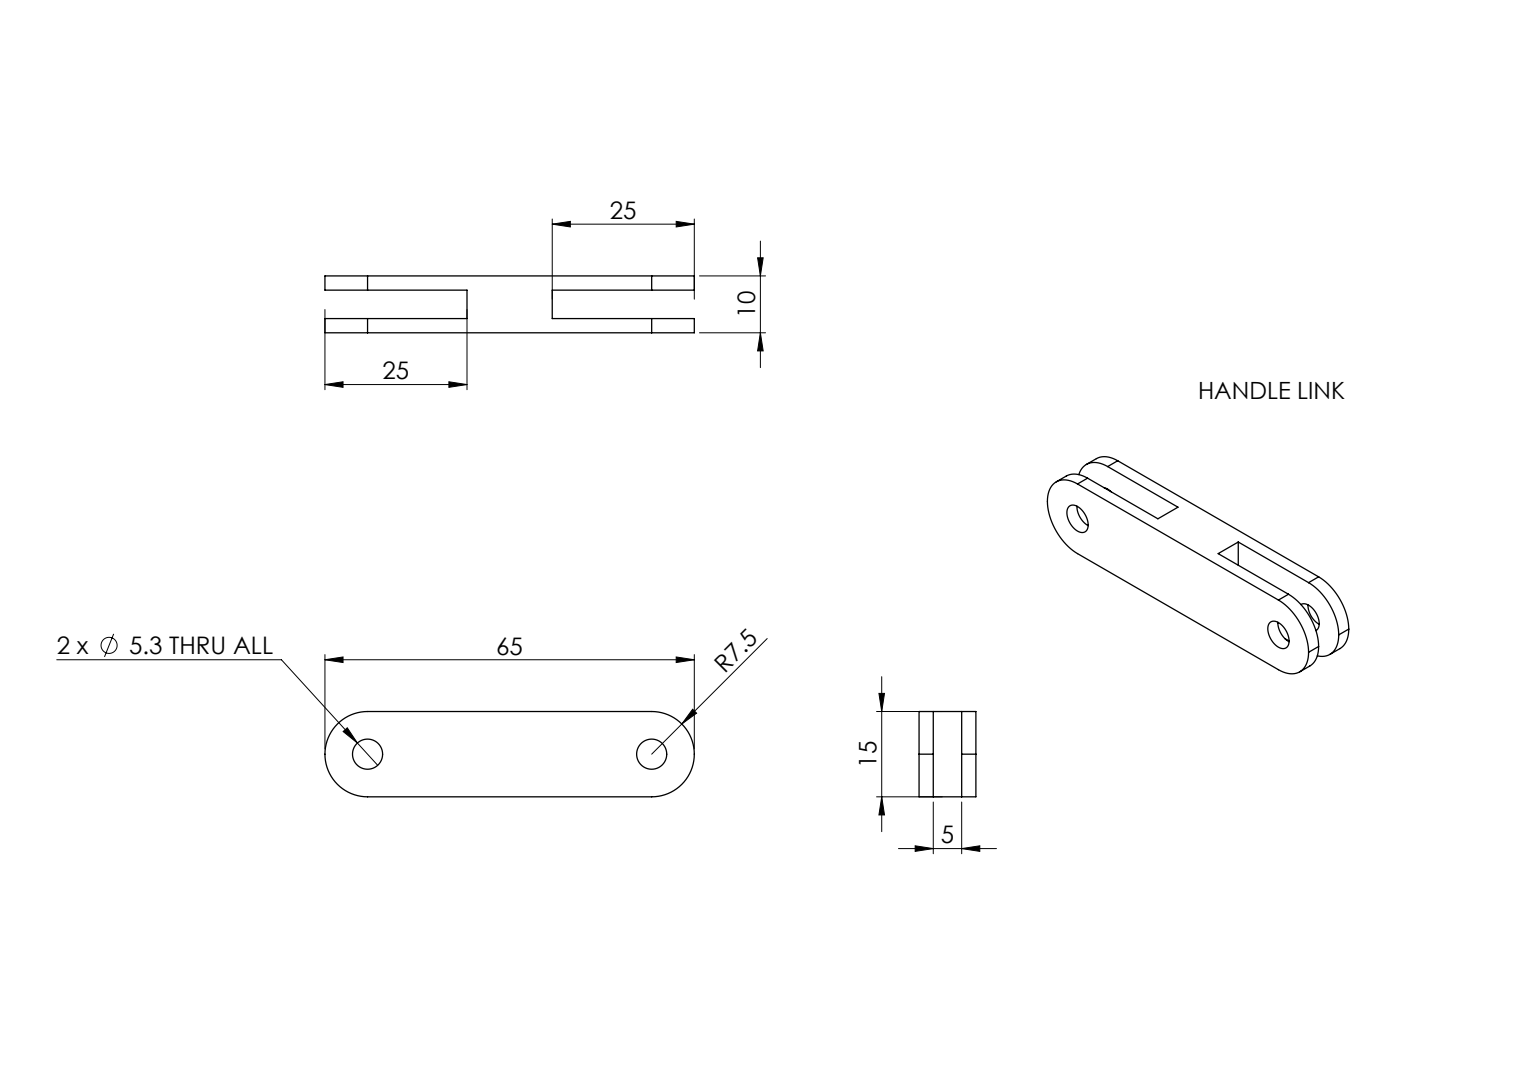
ISO-10303-21;
HEADER;
FILE_DESCRIPTION (('STEP AP214'),
    '1' );
FILE_NAME ('handle link.step',
    '2026-10-31T03:36:27',
    ( '' ),
    ( '' ),
    'SwSTEP 2.0',
    'SolidWorks 2026',
    '' );
FILE_SCHEMA (( 'AUTOMOTIVE_DESIGN' ));
ENDSEC;

DATA;
#3=ORIENTED_EDGE ( 'NONE', *, *, #2176, .T. ) ;
#65=ORIENTED_EDGE ( 'NONE', *, *, #28486, .T. ) ;
#85=DIRECTION ( 'NONE',  ( -0.000000000000000000, -0.000000000000000000, 1.000000000000000000 ) ) ;
#238=DIRECTION ( 'NONE',  ( -0.000000000000000000, -0.000000000000000000, 1.000000000000000000 ) ) ;
#278=CARTESIAN_POINT ( 'NONE',  ( -44.35000000000001563, 244.5000000000000000, -5.000000000000001776 ) ) ;
#331=DIRECTION ( 'NONE',  ( 0.000000000000000000, -0.000000000000000000, -1.000000000000000000 ) ) ;
#370=FACE_BOUND ( 'NONE', #668, .T. ) ;
#371=CARTESIAN_POINT ( 'NONE',  ( 0.3500000000000065281, 244.5000000000000000, 2.500000000000000000 ) ) ;
#373=DIRECTION ( 'NONE',  ( 0.000000000000000000, 0.000000000000000000, -1.000000000000000000 ) ) ;
#397=ORIENTED_EDGE ( 'NONE', *, *, #22014, .F. ) ;
#412=EDGE_CURVE ( 'NONE', #35111, #30074, #26288, .T. ) ;
#462=CIRCLE ( 'NONE', #24693, 2.649999999999992806 ) ;
#468=CARTESIAN_POINT ( 'NONE',  ( -54.50000000000000711, 244.5000000000000000, 5.000000000000000000 ) ) ;
#507=CARTESIAN_POINT ( 'NONE',  ( -47.00000000000000711, 244.5000000000000000, 5.000000000000000000 ) ) ;
#561=ORIENTED_EDGE ( 'NONE', *, *, #19014, .T. ) ;
#607=LINE ( 'NONE', #12176, #4334 ) ;
#668=EDGE_LOOP ( 'NONE', ( #20169, #31323 ) ) ;
#707=CIRCLE ( 'NONE', #4958, 2.649999999999991029 ) ;
#709=CARTESIAN_POINT ( 'NONE',  ( -49.64999999999999858, 244.5000000000000000, 5.000000000000000000 ) ) ;
#746=EDGE_CURVE ( 'NONE', #7363, #18087, #6969, .T. ) ;
#783=ORIENTED_EDGE ( 'NONE', *, *, #9463, .T. ) ;
#801=DIRECTION ( 'NONE',  ( 1.000000000000000000, 0.000000000000000000, 0.000000000000000000 ) ) ;
#814=CIRCLE ( 'NONE', #21430, 7.500000000000000000 ) ;
#882=ORIENTED_EDGE ( 'NONE', *, *, #5987, .T. ) ;
#914=LINE ( 'NONE', #15712, #11994 ) ;
#970=DIRECTION ( 'NONE',  ( -0.000000000000000000, -0.000000000000000000, 1.000000000000000000 ) ) ;
#1013=EDGE_CURVE ( 'NONE', #2263, #13555, #35585, .T. ) ;
#1029=LINE ( 'NONE', #4436, #15658 ) ;
#1046=ORIENTED_EDGE ( 'NONE', *, *, #23097, .F. ) ;
#1099=ORIENTED_EDGE ( 'NONE', *, *, #4077, .T. ) ;
#1123=CARTESIAN_POINT ( 'NONE',  ( 10.49999999999999645, 252.0000000000000000, -2.499999999999999556 ) ) ;
#1162=ORIENTED_EDGE ( 'NONE', *, *, #2683, .T. ) ;
#1167=DIRECTION ( 'NONE',  ( -0.000000000000000000, 1.000000000000000000, -0.000000000000000000 ) ) ;
#1216=FACE_OUTER_BOUND ( 'NONE', #2406, .T. ) ;
#1222=ORIENTED_EDGE ( 'NONE', *, *, #25857, .T. ) ;
#1245=FACE_OUTER_BOUND ( 'NONE', #30744, .T. ) ;
#1273=FACE_OUTER_BOUND ( 'NONE', #14565, .T. ) ;
#1385=VECTOR ( 'NONE', #16289, 1000.000000000000000 ) ;
#1454=CIRCLE ( 'NONE', #28104, 2.649999999999991029 ) ;
#1465=CARTESIAN_POINT ( 'NONE',  ( 2.999999999999997335, 244.5000000000000000, -2.499999999999999556 ) ) ;
#1472=CARTESIAN_POINT ( 'NONE',  ( 2.999999999999997335, 237.0000000000000000, 5.000000000000000000 ) ) ;
#1495=DIRECTION ( 'NONE',  ( 1.000000000000000000, 0.000000000000000000, 2.057406622567553763E-16 ) ) ;
#1510=CARTESIAN_POINT ( 'NONE',  ( 10.49999999999999467, 237.0000000000000000, -2.500000000000000000 ) ) ;
#1587=AXIS2_PLACEMENT_3D ( 'NONE', #16076, #33314, #36516 ) ;
#1637=ORIENTED_EDGE ( 'NONE', *, *, #15360, .F. ) ;
#1727=EDGE_LOOP ( 'NONE', ( #26472, #2358, #397, #19028 ) ) ;
#1742=CARTESIAN_POINT ( 'NONE',  ( -49.64999999999999147, 244.5000000000000000, 5.000000000000000888 ) ) ;
#1811=AXIS2_PLACEMENT_3D ( 'NONE', #26939, #970, #24112 ) ;
#1841=ORIENTED_EDGE ( 'NONE', *, *, #12878, .F. ) ;
#1883=LINE ( 'NONE', #4026, #2516 ) ;
#1921=( NAMED_UNIT ( * ) SI_UNIT ( $, .STERADIAN. ) SOLID_ANGLE_UNIT ( ) );
#1938=ORIENTED_EDGE ( 'NONE', *, *, #7640, .T. ) ;
#1964=CARTESIAN_POINT ( 'NONE',  ( -29.50000000000000711, 237.0000000000000000, -2.499999999999994671 ) ) ;
#1981=ORIENTED_EDGE ( 'NONE', *, *, #16185, .F. ) ;
#2017=CARTESIAN_POINT ( 'NONE',  ( -44.35000000000001563, 244.5000000000000000, 2.500000000000002220 ) ) ;
#2051=ADVANCED_FACE ( 'NONE', ( #370, #18586 ), #32779, .F. ) ;
#2131=LINE ( 'NONE', #10852, #3467 ) ;
#2150=LINE ( 'NONE', #1964, #13540 ) ;
#2175=CARTESIAN_POINT ( 'NONE',  ( 0.000000000000000000, 0.000000000000000000, 5.000000000000000000 ) ) ;
#2176=EDGE_CURVE ( 'NONE', #26234, #22829, #20863, .T. ) ;
#2188=EDGE_CURVE ( 'NONE', #6071, #13579, #21881, .T. ) ;
#2221=CARTESIAN_POINT ( 'NONE',  ( 10.49999999999999645, 252.0000000000000000, 2.500000000000000000 ) ) ;
#2263=VERTEX_POINT ( 'NONE', #3405 ) ;
#2308=ADVANCED_FACE ( 'NONE', ( #24627 ), #13071, .T. ) ;
#2330=FACE_OUTER_BOUND ( 'NONE', #20588, .T. ) ;
#2338=ORIENTED_EDGE ( 'NONE', *, *, #13660, .T. ) ;
#2358=ORIENTED_EDGE ( 'NONE', *, *, #23097, .T. ) ;
#2403=LINE ( 'NONE', #34432, #8203 ) ;
#2406=EDGE_LOOP ( 'NONE', ( #8339, #18616, #28272, #15794 ) ) ;
#2449=ORIENTED_EDGE ( 'NONE', *, *, #3200, .F. ) ;
#2509=CARTESIAN_POINT ( 'NONE',  ( 2.999999999999997335, 244.5000000000000000, 5.000000000000000000 ) ) ;
#2516=VECTOR ( 'NONE', #35484, 1000.000000000000000 ) ;
#2521=CARTESIAN_POINT ( 'NONE',  ( -14.50000000000000533, 237.0000000000000000, 2.500000000000000000 ) ) ;
#2546=ORIENTED_EDGE ( 'NONE', *, *, #30573, .F. ) ;
#2553=PLANE ( 'NONE',  #22436 ) ;
#2591=ORIENTED_EDGE ( 'NONE', *, *, #11969, .F. ) ;
#2625=CARTESIAN_POINT ( 'NONE',  ( -49.64999999999999858, 244.5000000000000000, -5.000000000000001776 ) ) ;
#2630=EDGE_LOOP ( 'NONE', ( #9394, #2897, #16899, #8425 ) ) ;
#2670=DIRECTION ( 'NONE',  ( 1.000000000000000000, 0.000000000000000000, 0.000000000000000000 ) ) ;
#2683=EDGE_CURVE ( 'NONE', #6822, #28262, #9292, .T. ) ;
#2705=DIRECTION ( 'NONE',  ( -1.000000000000000000, 0.000000000000000000, 0.000000000000000000 ) ) ;
#2707=ADVANCED_FACE ( 'NONE', ( #11238, #6257, #19795 ), #37195, .F. ) ;
#2831=VECTOR ( 'NONE', #373, 1000.000000000000000 ) ;
#2837=CARTESIAN_POINT ( 'NONE',  ( 2.999999999999997335, 237.0000000000000000, -5.000000000000000000 ) ) ;
#2875=ORIENTED_EDGE ( 'NONE', *, *, #11274, .F. ) ;
#2884=ORIENTED_EDGE ( 'NONE', *, *, #37146, .F. ) ;
#2897=ORIENTED_EDGE ( 'NONE', *, *, #6855, .F. ) ;
#2911=ORIENTED_EDGE ( 'NONE', *, *, #35826, .T. ) ;
#3007=ORIENTED_EDGE ( 'NONE', *, *, #16185, .T. ) ;
#3034=AXIS2_PLACEMENT_3D ( 'NONE', #30127, #4159, #1495 ) ;
#3054=ORIENTED_EDGE ( 'NONE', *, *, #7744, .T. ) ;
#3140=CARTESIAN_POINT ( 'NONE',  ( 5.649999999999991473, 244.5000000000000000, -5.000000000000001776 ) ) ;
#3174=LINE ( 'NONE', #11895, #3762 ) ;
#3191=ORIENTED_EDGE ( 'NONE', *, *, #13578, .T. ) ;
#3195=CIRCLE ( 'NONE', #34074, 2.649999999999992806 ) ;
#3200=EDGE_CURVE ( 'NONE', #9774, #8415, #9802, .T. ) ;
#3289=LINE ( 'NONE', #29442, #15484 ) ;
#3301=DIRECTION ( 'NONE',  ( 0.000000000000000000, 0.000000000000000000, -1.000000000000000000 ) ) ;
#3397=DIRECTION ( 'NONE',  ( -0.000000000000000000, -0.000000000000000000, 1.000000000000000000 ) ) ;
#3405=CARTESIAN_POINT ( 'NONE',  ( 5.649999999999985256, 244.5000000000000000, 5.000000000000000888 ) ) ;
#3467=VECTOR ( 'NONE', #11039, 1000.000000000000000 ) ;
#3543=EDGE_CURVE ( 'NONE', #22652, #25991, #3174, .T. ) ;
#3557=DIRECTION ( 'NONE',  ( 0.000000000000000000, -0.000000000000000000, -1.000000000000000000 ) ) ;
#3558=LINE ( 'NONE', #29135, #34671 ) ;
#3565=LINE ( 'NONE', #15128, #12722 ) ;
#3597=DIRECTION ( 'NONE',  ( 1.000000000000000000, 0.000000000000000000, 0.000000000000000000 ) ) ;
#3698=VERTEX_POINT ( 'NONE', #29326 ) ;
#3710=CARTESIAN_POINT ( 'NONE',  ( -47.00000000000000711, 237.0000000000000000, -5.000000000000000000 ) ) ;
#3718=CARTESIAN_POINT ( 'NONE',  ( -47.00000000000000711, 244.5000000000000000, 5.000000000000000000 ) ) ;
#3737=CARTESIAN_POINT ( 'NONE',  ( 2.999999999999997335, 244.5000000000000000, -2.499999999999999556 ) ) ;
#3762=VECTOR ( 'NONE', #35017, 1000.000000000000000 ) ;
#3778=DIRECTION ( 'NONE',  ( -1.000000000000000000, 0.000000000000000000, -0.000000000000000000 ) ) ;
#3907=CYLINDRICAL_SURFACE ( 'NONE', #14357, 2.649999999999992806 ) ;
#3929=CARTESIAN_POINT ( 'NONE',  ( -14.50000000000000533, 237.0000000000000000, 2.500000000000000000 ) ) ;
#3945=ORIENTED_EDGE ( 'NONE', *, *, #11087, .F. ) ;
#4026=CARTESIAN_POINT ( 'NONE',  ( 10.49999999999999645, 252.0000000000000000, 5.000000000000000000 ) ) ;
#4065=EDGE_CURVE ( 'NONE', #20125, #23018, #707, .T. ) ;
#4077=EDGE_CURVE ( 'NONE', #26234, #30347, #12463, .T. ) ;
#4138=ORIENTED_EDGE ( 'NONE', *, *, #3543, .T. ) ;
#4156=CARTESIAN_POINT ( 'NONE',  ( -47.00000000000000711, 244.5000000000000000, -2.499999999999997780 ) ) ;
#4159=DIRECTION ( 'NONE',  ( -2.057406622567553763E-16, 0.000000000000000000, 1.000000000000000000 ) ) ;
#4167=ORIENTED_EDGE ( 'NONE', *, *, #17535, .T. ) ;
#4206=FACE_OUTER_BOUND ( 'NONE', #5940, .T. ) ;
#4216=EDGE_LOOP ( 'NONE', ( #33261, #19684 ) ) ;
#4281=DIRECTION ( 'NONE',  ( -0.000000000000000000, -0.000000000000000000, 1.000000000000000000 ) ) ;
#4334=VECTOR ( 'NONE', #23750, 1000.000000000000000 ) ;
#4337=DIRECTION ( 'NONE',  ( 0.000000000000000000, 0.000000000000000000, -1.000000000000000000 ) ) ;
#4418=SHAPE_REPRESENTATION_RELATIONSHIP ( 'NONE' , 'NONE' ,  #16167, #5631 ) ;
#4436=CARTESIAN_POINT ( 'NONE',  ( -44.35000000000001563, 244.5000000000000000, 5.000000000000000000 ) ) ;
#4651=DIRECTION ( 'NONE',  ( 0.000000000000000000, 0.000000000000000000, 1.000000000000000000 ) ) ;
#4680=DIRECTION ( 'NONE',  ( 1.000000000000000000, 0.000000000000000000, 0.000000000000000000 ) ) ;
#4701=DIRECTION ( 'NONE',  ( 1.000000000000000000, 0.000000000000000000, 0.000000000000000000 ) ) ;
#4709=CARTESIAN_POINT ( 'NONE',  ( -14.50000000000000533, 237.0000000000000000, -2.500000000000000000 ) ) ;
#4714=AXIS2_PLACEMENT_3D ( 'NONE', #16980, #85, #37056 ) ;
#4765=AXIS2_PLACEMENT_3D ( 'NONE', #507, #31982, #5827 ) ;
#4839=CIRCLE ( 'NONE', #1811, 2.649999999999987477 ) ;
#4862=CARTESIAN_POINT ( 'NONE',  ( 0.3500000000000030864, 244.5000000000000000, -5.000000000000001776 ) ) ;
#4879=EDGE_LOOP ( 'NONE', ( #1046, #2449, #7578, #23453 ) ) ;
#4910=DIRECTION ( 'NONE',  ( -0.000000000000000000, -0.000000000000000000, 1.000000000000000000 ) ) ;
#4923=CARTESIAN_POINT ( 'NONE',  ( -29.50000000000000711, 252.0000000000000000, 5.000000000000000000 ) ) ;
#4937=CARTESIAN_POINT ( 'NONE',  ( -54.50000000000000711, 244.5000000000000000, -5.000000000000000000 ) ) ;
#4958=AXIS2_PLACEMENT_3D ( 'NONE', #3737, #3557, #15310 ) ;
#5133=LINE ( 'NONE', #19755, #11840 ) ;
#5159=PRESENTATION_STYLE_ASSIGNMENT (( #36626 ) ) ;
#5172=EDGE_CURVE ( 'NONE', #16919, #9886, #2150, .T. ) ;
#5199=EDGE_LOOP ( 'NONE', ( #10198, #34656, #29786, #28896 ) ) ;
#5275=CYLINDRICAL_SURFACE ( 'NONE', #14283, 2.649999999999992806 ) ;
#5328=LINE ( 'NONE', #11204, #35424 ) ;
#5352=CIRCLE ( 'NONE', #18095, 7.500000000000000000 ) ;
#5631=ADVANCED_BREP_SHAPE_REPRESENTATION ( '', ( #20231, #17215 ), #9874 ) ;
#5674=EDGE_CURVE ( 'NONE', #22116, #2263, #17878, .T. ) ;
#5688=CIRCLE ( 'NONE', #33550, 7.500000000000000000 ) ;
#5696=CARTESIAN_POINT ( 'NONE',  ( -47.00000000000000711, 244.5000000000000000, 2.500000000000001776 ) ) ;
#5734=DIRECTION ( 'NONE',  ( 0.000000000000000000, 0.000000000000000000, -1.000000000000000000 ) ) ;
#5827=DIRECTION ( 'NONE',  ( 1.000000000000000000, 0.000000000000000000, 0.000000000000000000 ) ) ;
#5877=ORIENTED_EDGE ( 'NONE', *, *, #30573, .T. ) ;
#5927=CIRCLE ( 'NONE', #9568, 7.500000000000000000 ) ;
#5940=EDGE_LOOP ( 'NONE', ( #8655, #3007, #28913, #16752 ) ) ;
#5961=EDGE_LOOP ( 'NONE', ( #12843, #35401, #13130, #13842 ) ) ;
#5987=EDGE_CURVE ( 'NONE', #22652, #8155, #814, .T. ) ;
#5990=EDGE_LOOP ( 'NONE', ( #24725, #23324 ) ) ;
#6018=FACE_OUTER_BOUND ( 'NONE', #27165, .T. ) ;
#6071=VERTEX_POINT ( 'NONE', #1742 ) ;
#6157=EDGE_CURVE ( 'NONE', #22829, #3698, #5328, .T. ) ;
#6253=DIRECTION ( 'NONE',  ( -0.000000000000000000, -0.000000000000000000, 1.000000000000000000 ) ) ;
#6257=FACE_BOUND ( 'NONE', #4216, .T. ) ;
#6346=EDGE_CURVE ( 'NONE', #37113, #27676, #28190, .T. ) ;
#6491=ORIENTED_EDGE ( 'NONE', *, *, #17296, .T. ) ;
#6492=CARTESIAN_POINT ( 'NONE',  ( 2.999999999999997335, 244.5000000000000000, 5.000000000000000000 ) ) ;
#6497=CARTESIAN_POINT ( 'NONE',  ( 5.649999999999987921, 244.5000000000000000, 5.000000000000000000 ) ) ;
#6522=( LENGTH_UNIT ( ) NAMED_UNIT ( * ) SI_UNIT ( .MILLI., .METRE. ) );
#6700=ORIENTED_EDGE ( 'NONE', *, *, #35373, .F. ) ;
#6773=DIRECTION ( 'NONE',  ( 0.000000000000000000, 0.000000000000000000, 1.000000000000000000 ) ) ;
#6796=EDGE_CURVE ( 'NONE', #8155, #18512, #36709, .T. ) ;
#6814=CARTESIAN_POINT ( 'NONE',  ( -47.00000000000000711, 244.5000000000000000, 5.000000000000000888 ) ) ;
#6822=VERTEX_POINT ( 'NONE', #17374 ) ;
#6855=EDGE_CURVE ( 'NONE', #19498, #35111, #14874, .T. ) ;
#6872=STYLED_ITEM ( 'NONE', ( #5159 ), #5631 ) ;
#6900=( NAMED_UNIT ( * ) PLANE_ANGLE_UNIT ( ) SI_UNIT ( $, .RADIAN. ) );
#6947=CARTESIAN_POINT ( 'NONE',  ( -47.00000000000000711, 244.5000000000000000, -2.499999999999997780 ) ) ;
#6969=LINE ( 'NONE', #24759, #12914 ) ;
#6988=DIRECTION ( 'NONE',  ( -0.000000000000000000, -0.000000000000000000, 1.000000000000000000 ) ) ;
#7001=CIRCLE ( 'NONE', #17894, 7.500000000000000000 ) ;
#7062=AXIS2_PLACEMENT_3D ( 'NONE', #31879, #19787, #8763 ) ;
#7110=VECTOR ( 'NONE', #36576, 1000.000000000000000 ) ;
#7176=CARTESIAN_POINT ( 'NONE',  ( 2.999999999999997335, 252.0000000000000000, -2.499999999999999556 ) ) ;
#7252=LINE ( 'NONE', #32828, #16365 ) ;
#7255=DIRECTION ( 'NONE',  ( 1.000000000000000000, 0.000000000000000000, 0.000000000000000000 ) ) ;
#7303=CARTESIAN_POINT ( 'NONE',  ( -54.50000000000000711, 244.5000000000000000, -2.499999999999996003 ) ) ;
#7315=DIRECTION ( 'NONE',  ( 1.000000000000000000, 0.000000000000000000, 1.636531581110199847E-16 ) ) ;
#7320=DIRECTION ( 'NONE',  ( -2.057406622567553763E-16, 0.000000000000000000, 1.000000000000000000 ) ) ;
#7354=CYLINDRICAL_SURFACE ( 'NONE', #21587, 2.649999999999991029 ) ;
#7363=VERTEX_POINT ( 'NONE', #32503 ) ;
#7364=VECTOR ( 'NONE', #35617, 1000.000000000000000 ) ;
#7379=AXIS2_PLACEMENT_3D ( 'NONE', #24131, #4910, #801 ) ;
#7529=AXIS2_PLACEMENT_3D ( 'NONE', #20789, #9780, #12624 ) ;
#7541=DIRECTION ( 'NONE',  ( -1.000000000000000000, 0.000000000000000000, 0.000000000000000000 ) ) ;
#7578=ORIENTED_EDGE ( 'NONE', *, *, #20721, .T. ) ;
#7588=CIRCLE ( 'NONE', #34813, 2.649999999999992806 ) ;
#7623=( LENGTH_UNIT ( ) NAMED_UNIT ( * ) SI_UNIT ( .MILLI., .METRE. ) );
#7640=EDGE_CURVE ( 'NONE', #22958, #37113, #5688, .T. ) ;
#7744=EDGE_CURVE ( 'NONE', #9886, #19776, #29044, .T. ) ;
#7861=LINE ( 'NONE', #30983, #27840 ) ;
#7973=AXIS2_PLACEMENT_3D ( 'NONE', #28857, #238, #14843 ) ;
#8154=EDGE_LOOP ( 'NONE', ( #28821, #2546, #20599, #10061, #36654 ) ) ;
#8155=VERTEX_POINT ( 'NONE', #2837 ) ;
#8174=DIRECTION ( 'NONE',  ( 0.000000000000000000, 0.000000000000000000, 1.000000000000000000 ) ) ;
#8203=VECTOR ( 'NONE', #29101, 1000.000000000000000 ) ;
#8279=DIRECTION ( 'NONE',  ( -1.000000000000000000, 0.000000000000000000, 0.000000000000000000 ) ) ;
#8299=EDGE_CURVE ( 'NONE', #18605, #13555, #34233, .T. ) ;
#8339=ORIENTED_EDGE ( 'NONE', *, *, #19918, .F. ) ;
#8341=CARTESIAN_POINT ( 'NONE',  ( 10.49999999999999467, 237.0000000000000000, -2.500000000000000000 ) ) ;
#8375=DIRECTION ( 'NONE',  ( -0.000000000000000000, -0.000000000000000000, 1.000000000000000000 ) ) ;
#8395=VERTEX_POINT ( 'NONE', #2017 ) ;
#8415=VERTEX_POINT ( 'NONE', #4862 ) ;
#8425=ORIENTED_EDGE ( 'NONE', *, *, #25413, .T. ) ;
#8464=DIRECTION ( 'NONE',  ( -0.000000000000000000, -0.000000000000000000, 1.000000000000000000 ) ) ;
#8536=CARTESIAN_POINT ( 'NONE',  ( 2.999999999999997335, 252.0000000000000000, 5.000000000000000000 ) ) ;
#8545=EDGE_LOOP ( 'NONE', ( #21634, #17320, #12168, #8842 ) ) ;
#8594=VERTEX_POINT ( 'NONE', #468 ) ;
#8655=ORIENTED_EDGE ( 'NONE', *, *, #31634, .F. ) ;
#8763=DIRECTION ( 'NONE',  ( -1.000000000000000000, 0.000000000000000000, 0.000000000000000000 ) ) ;
#8778=CARTESIAN_POINT ( 'NONE',  ( 2.999999999999997335, 244.5000000000000000, 5.000000000000000000 ) ) ;
#8786=CARTESIAN_POINT ( 'NONE',  ( 2.999999999999997335, 244.5000000000000000, 5.000000000000000000 ) ) ;
#8797=ORIENTED_EDGE ( 'NONE', *, *, #9372, .F. ) ;
#8800=FACE_OUTER_BOUND ( 'NONE', #5199, .T. ) ;
#8842=ORIENTED_EDGE ( 'NONE', *, *, #25857, .F. ) ;
#8902=ADVANCED_FACE ( 'NONE', ( #1216 ), #12983, .T. ) ;
#8907=AXIS2_PLACEMENT_3D ( 'NONE', #21819, #22562, #28052 ) ;
#9029=DIRECTION ( 'NONE',  ( -1.000000000000000000, -0.000000000000000000, -0.000000000000000000 ) ) ;
#9107=( GEOMETRIC_REPRESENTATION_CONTEXT ( 3 ) GLOBAL_UNCERTAINTY_ASSIGNED_CONTEXT ( ( #30949 ) ) GLOBAL_UNIT_ASSIGNED_CONTEXT ( ( #7623, #16529, #1921 ) ) REPRESENTATION_CONTEXT ( 'NONE', 'WORKASPACE' ) );
#9234=EDGE_CURVE ( 'NONE', #13579, #6071, #18891, .T. ) ;
#9292=LINE ( 'NONE', #2521, #2831 ) ;
#9372=EDGE_CURVE ( 'NONE', #8155, #25296, #607, .T. ) ;
#9384=ADVANCED_FACE ( 'NONE', ( #32455 ), #34735, .T. ) ;
#9394=ORIENTED_EDGE ( 'NONE', *, *, #412, .F. ) ;
#9434=LINE ( 'NONE', #29327, #32953 ) ;
#9463=EDGE_CURVE ( 'NONE', #27676, #12668, #1883, .T. ) ;
#9509=ADVANCED_FACE ( 'NONE', ( #24320 ), #12565, .F. ) ;
#9528=DIRECTION ( 'NONE',  ( 0.000000000000000000, 0.000000000000000000, -1.000000000000000000 ) ) ;
#9534=CARTESIAN_POINT ( 'NONE',  ( -44.35000000000001563, 244.5000000000000000, -2.499999999999997335 ) ) ;
#9568=AXIS2_PLACEMENT_3D ( 'NONE', #33173, #16493, #25006 ) ;
#9774=VERTEX_POINT ( 'NONE', #3140 ) ;
#9780=DIRECTION ( 'NONE',  ( 2.057406622567553763E-16, -0.000000000000000000, -1.000000000000000000 ) ) ;
#9802=CIRCLE ( 'NONE', #18915, 2.649999999999994582 ) ;
#9814=CARTESIAN_POINT ( 'NONE',  ( -49.64999999999999858, 244.5000000000000000, 2.500000000000001332 ) ) ;
#9874=( GEOMETRIC_REPRESENTATION_CONTEXT ( 3 ) GLOBAL_UNCERTAINTY_ASSIGNED_CONTEXT ( ( #30177 ) ) GLOBAL_UNIT_ASSIGNED_CONTEXT ( ( #6522, #6900, #26793 ) ) REPRESENTATION_CONTEXT ( 'NONE', 'WORKASPACE' ) );
#9886=VERTEX_POINT ( 'NONE', #36279 ) ;
#9963=DIRECTION ( 'NONE',  ( -2.057406622567553763E-16, 0.000000000000000000, 1.000000000000000000 ) ) ;
#9964=CARTESIAN_POINT ( 'NONE',  ( -54.50000000000000711, 244.5000000000000000, 2.500000000000000000 ) ) ;
#9998=CARTESIAN_POINT ( 'NONE',  ( 2.999999999999997335, 244.5000000000000000, -5.000000000000000000 ) ) ;
#10061=ORIENTED_EDGE ( 'NONE', *, *, #11969, .T. ) ;
#10109=ADVANCED_FACE ( 'NONE', ( #30533, #28786 ), #26640, .F. ) ;
#10126=EDGE_LOOP ( 'NONE', ( #37387, #24919, #12050, #3054 ) ) ;
#10188=ORIENTED_EDGE ( 'NONE', *, *, #5172, .F. ) ;
#10198=ORIENTED_EDGE ( 'NONE', *, *, #8299, .F. ) ;
#10201=PRODUCT_DEFINITION ( 'UNKNOWN', '', #22055, #26269 ) ;
#10259=EDGE_LOOP ( 'NONE', ( #16320, #36183, #33664, #12933 ) ) ;
#10274=CARTESIAN_POINT ( 'NONE',  ( 2.999999999999997335, 244.5000000000000000, -5.000000000000000000 ) ) ;
#10343=CARTESIAN_POINT ( 'NONE',  ( -47.00000000000000711, 244.5000000000000000, 2.500000000000001776 ) ) ;
#10463=DIRECTION ( 'NONE',  ( 1.000000000000000000, 0.000000000000000000, 0.000000000000000000 ) ) ;
#10464=EDGE_LOOP ( 'NONE', ( #10725, #31213, #2875, #18973 ) ) ;
#10501=VECTOR ( 'NONE', #18451, 1000.000000000000000 ) ;
#10560=DIRECTION ( 'NONE',  ( 0.000000000000000000, -0.000000000000000000, -1.000000000000000000 ) ) ;
#10620=ORIENTED_EDGE ( 'NONE', *, *, #14204, .T. ) ;
#10647=CARTESIAN_POINT ( 'NONE',  ( -47.00000000000000711, 244.5000000000000000, -5.000000000000001776 ) ) ;
#10665=( LENGTH_UNIT ( ) NAMED_UNIT ( * ) SI_UNIT ( .MILLI., .METRE. ) );
#10704=ORIENTED_EDGE ( 'NONE', *, *, #412, .T. ) ;
#10725=ORIENTED_EDGE ( 'NONE', *, *, #24289, .F. ) ;
#10779=ADVANCED_FACE ( 'NONE', ( #33119 ), #18350, .T. ) ;
#10821=CYLINDRICAL_SURFACE ( 'NONE', #24614, 7.500000000000000000 ) ;
#10852=CARTESIAN_POINT ( 'NONE',  ( 10.49999999999999645, 252.0000000000000000, 2.500000000000013323 ) ) ;
#10853=( NAMED_UNIT ( * ) SI_UNIT ( $, .STERADIAN. ) SOLID_ANGLE_UNIT ( ) );
#10934=CARTESIAN_POINT ( 'NONE',  ( 2.999999999999997335, 237.0000000000000000, 5.000000000000000000 ) ) ;
#10935=AXIS2_PLACEMENT_3D ( 'NONE', #10343, #7320, #18521 ) ;
#10991=EDGE_CURVE ( 'NONE', #30074, #14298, #3195, .T. ) ;
#11006=CARTESIAN_POINT ( 'NONE',  ( -47.00000000000000711, 244.5000000000000000, 5.000000000000000000 ) ) ;
#11008=ADVANCED_FACE ( 'NONE', ( #27276 ), #35613, .T. ) ;
#11039=DIRECTION ( 'NONE',  ( -1.000000000000000000, 0.000000000000000000, -2.057406622567553763E-16 ) ) ;
#11068=DIRECTION ( 'NONE',  ( 1.000000000000000000, 0.000000000000000000, 2.057406622567553516E-16 ) ) ;
#11087=EDGE_CURVE ( 'NONE', #28262, #26234, #30692, .T. ) ;
#11115=CARTESIAN_POINT ( 'NONE',  ( -29.50000000000000711, 237.0000000000000000, -2.499999999999994671 ) ) ;
#11189=FACE_OUTER_BOUND ( 'NONE', #8545, .T. ) ;
#11204=CARTESIAN_POINT ( 'NONE',  ( 2.999999999999997335, 252.0000000000000000, -5.000000000000000000 ) ) ;
#11238=FACE_BOUND ( 'NONE', #18843, .T. ) ;
#11266=ORIENTED_EDGE ( 'NONE', *, *, #746, .T. ) ;
#11274=EDGE_CURVE ( 'NONE', #8594, #36846, #5352, .T. ) ;
#11293=CARTESIAN_POINT ( 'NONE',  ( -54.50000000000000711, 237.0000000000000000, -2.500000000000000000 ) ) ;
#11434=DIRECTION ( 'NONE',  ( -1.000000000000000000, 0.000000000000000000, -0.000000000000000000 ) ) ;
#11488=ORIENTED_EDGE ( 'NONE', *, *, #19918, .T. ) ;
#11511=AXIS2_PLACEMENT_3D ( 'NONE', #25828, #14459, #26014 ) ;
#11527=DIRECTION ( 'NONE',  ( 0.000000000000000000, -1.000000000000000000, 0.000000000000000000 ) ) ;
#11552=EDGE_CURVE ( 'NONE', #12668, #8594, #27770, .T. ) ;
#11840=VECTOR ( 'NONE', #34683, 1000.000000000000000 ) ;
#11895=CARTESIAN_POINT ( 'NONE',  ( 10.49999999999999645, 244.5000000000000000, 5.000000000000000000 ) ) ;
#11907=DIRECTION ( 'NONE',  ( -1.000000000000000000, 0.000000000000000000, 0.000000000000000000 ) ) ;
#11969=EDGE_CURVE ( 'NONE', #16035, #16919, #19658, .T. ) ;
#11994=VECTOR ( 'NONE', #33141, 1000.000000000000000 ) ;
#12050=ORIENTED_EDGE ( 'NONE', *, *, #5172, .T. ) ;
#12077=DIRECTION ( 'NONE',  ( -0.000000000000000000, -0.000000000000000000, 1.000000000000000000 ) ) ;
#12119=LINE ( 'NONE', #23886, #15170 ) ;
#12121=LINE ( 'NONE', #26712, #32691 ) ;
#12168=ORIENTED_EDGE ( 'NONE', *, *, #11552, .F. ) ;
#12176=CARTESIAN_POINT ( 'NONE',  ( 10.49999999999999645, 237.0000000000000000, -5.000000000000000000 ) ) ;
#12331=ORIENTED_EDGE ( 'NONE', *, *, #5987, .F. ) ;
#12463=LINE ( 'NONE', #24032, #27344 ) ;
#12497=DIRECTION ( 'NONE',  ( -1.000000000000000000, 0.000000000000000000, 0.000000000000000000 ) ) ;
#12565=CYLINDRICAL_SURFACE ( 'NONE', #7379, 2.649999999999992806 ) ;
#12624=DIRECTION ( 'NONE',  ( 1.000000000000000000, 0.000000000000000000, 2.312964634635742957E-16 ) ) ;
#12628=FACE_BOUND ( 'NONE', #5990, .T. ) ;
#12644=DIRECTION ( 'NONE',  ( -0.000000000000000000, -0.000000000000000000, 1.000000000000000000 ) ) ;
#12648=FACE_OUTER_BOUND ( 'NONE', #36783, .T. ) ;
#12668=VERTEX_POINT ( 'NONE', #30027 ) ;
#12676=CARTESIAN_POINT ( 'NONE',  ( -14.50000000000000533, 237.0000000000000000, -2.500000000000000000 ) ) ;
#12689=DIRECTION ( 'NONE',  ( 1.000000000000000000, 0.000000000000000000, 2.057406622567553763E-16 ) ) ;
#12722=VECTOR ( 'NONE', #19809, 1000.000000000000000 ) ;
#12739=CARTESIAN_POINT ( 'NONE',  ( -47.00000000000000711, 252.0000000000000000, -2.499999999999997780 ) ) ;
#12747=CIRCLE ( 'NONE', #30907, 7.500000000000000000 ) ;
#12762=CIRCLE ( 'NONE', #19462, 2.649999999999991029 ) ;
#12825=ORIENTED_EDGE ( 'NONE', *, *, #4077, .F. ) ;
#12843=ORIENTED_EDGE ( 'NONE', *, *, #37247, .F. ) ;
#12878=EDGE_CURVE ( 'NONE', #19498, #14298, #1029, .T. ) ;
#12895=AXIS2_PLACEMENT_3D ( 'NONE', #30508, #16104, #24441 ) ;
#12914=VECTOR ( 'NONE', #35943, 1000.000000000000000 ) ;
#12933=ORIENTED_EDGE ( 'NONE', *, *, #6157, .F. ) ;
#12983=CYLINDRICAL_SURFACE ( 'NONE', #13585, 7.500000000000000000 ) ;
#13070=FACE_BOUND ( 'NONE', #24873, .T. ) ;
#13071=CYLINDRICAL_SURFACE ( 'NONE', #28853, 7.500000000000000000 ) ;
#13130=ORIENTED_EDGE ( 'NONE', *, *, #35419, .F. ) ;
#13172=CARTESIAN_POINT ( 'NONE',  ( 2.999999999999997335, 244.5000000000000000, -2.499999999999999556 ) ) ;
#13247=CARTESIAN_POINT ( 'NONE',  ( 2.999999999999997335, 244.5000000000000000, -5.000000000000001776 ) ) ;
#13338=CIRCLE ( 'NONE', #34519, 7.500000000000000000 ) ;
#13376=DIRECTION ( 'NONE',  ( -0.000000000000000000, 0.000000000000000000, 1.000000000000000000 ) ) ;
#13456=FACE_OUTER_BOUND ( 'NONE', #31538, .T. ) ;
#13540=VECTOR ( 'NONE', #27934, 1000.000000000000000 ) ;
#13552=ORIENTED_EDGE ( 'NONE', *, *, #18146, .F. ) ;
#13554=ORIENTED_EDGE ( 'NONE', *, *, #2188, .T. ) ;
#13555=VERTEX_POINT ( 'NONE', #23662 ) ;
#13578=EDGE_CURVE ( 'NONE', #21882, #6071, #14942, .T. ) ;
#13579=VERTEX_POINT ( 'NONE', #21019 ) ;
#13585=AXIS2_PLACEMENT_3D ( 'NONE', #21706, #18495, #33256 ) ;
#13595=CARTESIAN_POINT ( 'NONE',  ( 0.3500000000000065281, 244.5000000000000000, 5.000000000000000000 ) ) ;
#13623=EDGE_CURVE ( 'NONE', #16919, #20032, #3565, .T. ) ;
#13660=EDGE_CURVE ( 'NONE', #36103, #9886, #7861, .T. ) ;
#13757=DIRECTION ( 'NONE',  ( 1.000000000000000000, 0.000000000000000000, 0.000000000000000000 ) ) ;
#13836=DIRECTION ( 'NONE',  ( -1.000000000000000000, -0.000000000000000000, -0.000000000000000000 ) ) ;
#13842=ORIENTED_EDGE ( 'NONE', *, *, #6346, .F. ) ;
#13877=DIRECTION ( 'NONE',  ( -0.000000000000000000, -0.000000000000000000, 1.000000000000000000 ) ) ;
#13888=EDGE_CURVE ( 'NONE', #13555, #2263, #4839, .T. ) ;
#13901=DIRECTION ( 'NONE',  ( 0.000000000000000000, -0.000000000000000000, -1.000000000000000000 ) ) ;
#13909=ORIENTED_EDGE ( 'NONE', *, *, #9234, .F. ) ;
#13933=ORIENTED_EDGE ( 'NONE', *, *, #25413, .F. ) ;
#14204=EDGE_CURVE ( 'NONE', #3698, #7363, #28487, .T. ) ;
#14283=AXIS2_PLACEMENT_3D ( 'NONE', #20816, #12077, #20628 ) ;
#14298=VERTEX_POINT ( 'NONE', #9534 ) ;
#14357=AXIS2_PLACEMENT_3D ( 'NONE', #3718, #4281, #35929 ) ;
#14459=DIRECTION ( 'NONE',  ( 0.000000000000000000, -0.000000000000000000, -1.000000000000000000 ) ) ;
#14462=DIRECTION ( 'NONE',  ( -1.000000000000000000, 0.000000000000000000, -0.000000000000000000 ) ) ;
#14474=ORIENTED_EDGE ( 'NONE', *, *, #35373, .T. ) ;
#14483=ORIENTED_EDGE ( 'NONE', *, *, #2176, .F. ) ;
#14529=ORIENTED_EDGE ( 'NONE', *, *, #9234, .T. ) ;
#14565=EDGE_LOOP ( 'NONE', ( #6491, #19954, #16359, #19403 ) ) ;
#14596=DIRECTION ( 'NONE',  ( 1.000000000000000000, 0.000000000000000000, 0.000000000000000000 ) ) ;
#14646=DIRECTION ( 'NONE',  ( 0.000000000000000000, -0.000000000000000000, -1.000000000000000000 ) ) ;
#14655=EDGE_LOOP ( 'NONE', ( #21402, #20315, #28222, #24098, #23575 ) ) ;
#14738=ORIENTED_EDGE ( 'NONE', *, *, #26044, .F. ) ;
#14782=CYLINDRICAL_SURFACE ( 'NONE', #15195, 2.649999999999991029 ) ;
#14791=DIRECTION ( 'NONE',  ( 1.000000000000000000, 0.000000000000000000, 0.000000000000000000 ) ) ;
#14843=DIRECTION ( 'NONE',  ( 1.000000000000000000, 0.000000000000000000, 0.000000000000000000 ) ) ;
#14861=CARTESIAN_POINT ( 'NONE',  ( 2.999999999999997335, 244.5000000000000000, 5.000000000000000000 ) ) ;
#14874=CIRCLE ( 'NONE', #29396, 2.649999999999992806 ) ;
#14942=LINE ( 'NONE', #709, #24810 ) ;
#14951=ORIENTED_EDGE ( 'NONE', *, *, #19014, .F. ) ;
#15034=VECTOR ( 'NONE', #35027, 1000.000000000000000 ) ;
#15128=CARTESIAN_POINT ( 'NONE',  ( -29.50000000000000711, 237.0000000000000000, -2.499999999999994671 ) ) ;
#15140=ADVANCED_FACE ( 'NONE', ( #25610 ), #34328, .T. ) ;
#15170=VECTOR ( 'NONE', #6253, 1000.000000000000000 ) ;
#15195=AXIS2_PLACEMENT_3D ( 'NONE', #22758, #3397, #37322 ) ;
#15310=DIRECTION ( 'NONE',  ( -1.000000000000000000, 0.000000000000000000, 0.000000000000000000 ) ) ;
#15311=PLANE ( 'NONE',  #19040 ) ;
#15314=CARTESIAN_POINT ( 'NONE',  ( 10.49999999999999645, 244.5000000000000000, 2.500000000000000000 ) ) ;
#15360=EDGE_CURVE ( 'NONE', #31488, #30489, #12747, .T. ) ;
#15484=VECTOR ( 'NONE', #35123, 1000.000000000000000 ) ;
#15634=AXIS2_PLACEMENT_3D ( 'NONE', #30524, #33731, #36562 ) ;
#15658=VECTOR ( 'NONE', #35527, 1000.000000000000000 ) ;
#15712=CARTESIAN_POINT ( 'NONE',  ( -47.00000000000000711, 237.0000000000000000, 5.000000000000000000 ) ) ;
#15726=DIRECTION ( 'NONE',  ( 1.000000000000000000, 0.000000000000000000, 1.636531581110199847E-16 ) ) ;
#15782=UNCERTAINTY_MEASURE_WITH_UNIT (LENGTH_MEASURE( 1.000000000000000082E-05 ), #10665, 'distance_accuracy_value', 'NONE');
#15794=ORIENTED_EDGE ( 'NONE', *, *, #19765, .F. ) ;
#15827=EDGE_CURVE ( 'NONE', #8395, #21882, #33932, .T. ) ;
#15907=ADVANCED_FACE ( 'NONE', ( #12628, #19454, #27780 ), #2553, .T. ) ;
#15970=ORIENTED_EDGE ( 'NONE', *, *, #6796, .F. ) ;
#16035=VERTEX_POINT ( 'NONE', #26794 ) ;
#16047=CARTESIAN_POINT ( 'NONE',  ( 0.000000000000000000, 0.000000000000000000, 0.000000000000000000 ) ) ;
#16076=CARTESIAN_POINT ( 'NONE',  ( 2.999999999999997335, 244.5000000000000000, 5.000000000000000000 ) ) ;
#16104=DIRECTION ( 'NONE',  ( 0.000000000000000000, 0.000000000000000000, -1.000000000000000000 ) ) ;
#16120=LINE ( 'NONE', #1510, #31968 ) ;
#16167=SHAPE_REPRESENTATION ( 'handle link', ( #17215 ), #9874 ) ;
#16185=EDGE_CURVE ( 'NONE', #30240, #31488, #13338, .T. ) ;
#16263=EDGE_LOOP ( 'NONE', ( #2911, #1637, #1981, #4167, #21374 ) ) ;
#16273=VECTOR ( 'NONE', #19127, 1000.000000000000000 ) ;
#16289=DIRECTION ( 'NONE',  ( -0.000000000000000000, 1.000000000000000000, -0.000000000000000000 ) ) ;
#16320=ORIENTED_EDGE ( 'NONE', *, *, #26959, .F. ) ;
#16359=ORIENTED_EDGE ( 'NONE', *, *, #13888, .T. ) ;
#16365=VECTOR ( 'NONE', #9528, 1000.000000000000000 ) ;
#16374=CARTESIAN_POINT ( 'NONE',  ( 2.999999999999997335, 237.0000000000000000, 2.500000000000000000 ) ) ;
#16445=PLANE ( 'NONE',  #23251 ) ;
#16480=PLANE ( 'NONE',  #3034 ) ;
#16493=DIRECTION ( 'NONE',  ( 2.057406622567553763E-16, -0.000000000000000000, -1.000000000000000000 ) ) ;
#16519=DIRECTION ( 'NONE',  ( 0.000000000000000000, 0.000000000000000000, -1.000000000000000000 ) ) ;
#16529=( NAMED_UNIT ( * ) PLANE_ANGLE_UNIT ( ) SI_UNIT ( $, .RADIAN. ) );
#16538=FACE_OUTER_BOUND ( 'NONE', #4879, .T. ) ;
#16539=ORIENTED_EDGE ( 'NONE', *, *, #23362, .F. ) ;
#16742=ORIENTED_EDGE ( 'NONE', *, *, #35419, .T. ) ;
#16752=ORIENTED_EDGE ( 'NONE', *, *, #7640, .F. ) ;
#16815=CARTESIAN_POINT ( 'NONE',  ( 2.999999999999997335, 237.0000000000000000, 5.000000000000000000 ) ) ;
#16853=DIRECTION ( 'NONE',  ( -0.000000000000000000, 0.000000000000000000, 1.000000000000000000 ) ) ;
#16899=ORIENTED_EDGE ( 'NONE', *, *, #12878, .T. ) ;
#16904=DIRECTION ( 'NONE',  ( 0.000000000000000000, 0.000000000000000000, -1.000000000000000000 ) ) ;
#16919=VERTEX_POINT ( 'NONE', #25960 ) ;
#16937=DIRECTION ( 'NONE',  ( -0.000000000000000000, 0.000000000000000000, 1.000000000000000000 ) ) ;
#16980=CARTESIAN_POINT ( 'NONE',  ( 2.999999999999997335, 244.5000000000000000, 5.000000000000000888 ) ) ;
#17064=AXIS2_PLACEMENT_3D ( 'NONE', #8778, #28668, #2705 ) ;
#17111=ADVANCED_FACE ( 'NONE', ( #17632 ), #14782, .F. ) ;
#17141=ORIENTED_EDGE ( 'NONE', *, *, #6346, .T. ) ;
#17215=AXIS2_PLACEMENT_3D ( 'NONE', #16047, #4651, #19645 ) ;
#17296=EDGE_CURVE ( 'NONE', #22116, #18605, #12762, .T. ) ;
#17320=ORIENTED_EDGE ( 'NONE', *, *, #27448, .F. ) ;
#17349=AXIS2_PLACEMENT_3D ( 'NONE', #1465, #10560, #7541 ) ;
#17374=CARTESIAN_POINT ( 'NONE',  ( -14.50000000000000533, 237.0000000000000000, 2.500000000000000000 ) ) ;
#17467=VECTOR ( 'NONE', #31201, 1000.000000000000000 ) ;
#17535=EDGE_CURVE ( 'NONE', #30240, #6822, #20227, .T. ) ;
#17632=FACE_OUTER_BOUND ( 'NONE', #1727, .T. ) ;
#17637=VECTOR ( 'NONE', #1167, 1000.000000000000000 ) ;
#17779=EDGE_LOOP ( 'NONE', ( #6700, #15970, #12331, #4138 ) ) ;
#17878=LINE ( 'NONE', #6497, #10501 ) ;
#17894=AXIS2_PLACEMENT_3D ( 'NONE', #5696, #31666, #28815 ) ;
#18016=CARTESIAN_POINT ( 'NONE',  ( -47.00000000000000711, 252.0000000000000000, 2.500000000000001776 ) ) ;
#18041=ORIENTED_EDGE ( 'NONE', *, *, #37182, .T. ) ;
#18043=ORIENTED_EDGE ( 'NONE', *, *, #6796, .T. ) ;
#18066=DIRECTION ( 'NONE',  ( 0.000000000000000000, 0.000000000000000000, -1.000000000000000000 ) ) ;
#18087=VERTEX_POINT ( 'NONE', #12739 ) ;
#18095=AXIS2_PLACEMENT_3D ( 'NONE', #25365, #33897, #37289 ) ;
#18146=EDGE_CURVE ( 'NONE', #6822, #30347, #29982, .T. ) ;
#18217=DIRECTION ( 'NONE',  ( 1.000000000000000000, 0.000000000000000000, 0.000000000000000000 ) ) ;
#18350=PLANE ( 'NONE',  #18947 ) ;
#18366=ORIENTED_EDGE ( 'NONE', *, *, #9372, .T. ) ;
#18451=DIRECTION ( 'NONE',  ( -0.000000000000000000, -0.000000000000000000, 1.000000000000000000 ) ) ;
#18474=SURFACE_STYLE_FILL_AREA ( #32852 ) ;
#18495=DIRECTION ( 'NONE',  ( 0.000000000000000000, 0.000000000000000000, -1.000000000000000000 ) ) ;
#18512=VERTEX_POINT ( 'NONE', #30560 ) ;
#18521=DIRECTION ( 'NONE',  ( 1.000000000000000000, 0.000000000000000000, 1.636531581110199847E-16 ) ) ;
#18586=FACE_OUTER_BOUND ( 'NONE', #14655, .T. ) ;
#18605=VERTEX_POINT ( 'NONE', #371 ) ;
#18616=ORIENTED_EDGE ( 'NONE', *, *, #34724, .T. ) ;
#18806=AXIS2_PLACEMENT_3D ( 'NONE', #28632, #25980, #2670 ) ;
#18843=EDGE_LOOP ( 'NONE', ( #35272, #65 ) ) ;
#18862=AXIS2_PLACEMENT_3D ( 'NONE', #26906, #27099, #12689 ) ;
#18891=CIRCLE ( 'NONE', #7973, 2.649999999999985700 ) ;
#18903=SHAPE_DEFINITION_REPRESENTATION ( #25892, #16167 ) ;
#18915=AXIS2_PLACEMENT_3D ( 'NONE', #25372, #28216, #19710 ) ;
#18947=AXIS2_PLACEMENT_3D ( 'NONE', #3929, #30313, #4337 ) ;
#18973=ORIENTED_EDGE ( 'NONE', *, *, #27448, .T. ) ;
#19014=EDGE_CURVE ( 'NONE', #22958, #36846, #12121, .T. ) ;
#19019=VERTEX_POINT ( 'NONE', #18016 ) ;
#19028=ORIENTED_EDGE ( 'NONE', *, *, #20721, .F. ) ;
#19034=VECTOR ( 'NONE', #28675, 1000.000000000000000 ) ;
#19040=AXIS2_PLACEMENT_3D ( 'NONE', #20447, #11527, #23096 ) ;
#19127=DIRECTION ( 'NONE',  ( 1.000000000000000000, 0.000000000000000000, 0.000000000000000000 ) ) ;
#19210=AXIS2_PLACEMENT_3D ( 'NONE', #22811, #16937, #14791 ) ;
#19319=LINE ( 'NONE', #2221, #16273 ) ;
#19390=DIRECTION ( 'NONE',  ( 0.000000000000000000, -0.000000000000000000, -1.000000000000000000 ) ) ;
#19403=ORIENTED_EDGE ( 'NONE', *, *, #5674, .F. ) ;
#19454=FACE_BOUND ( 'NONE', #31295, .T. ) ;
#19462=AXIS2_PLACEMENT_3D ( 'NONE', #20853, #32771, #12497 ) ;
#19485=CARTESIAN_POINT ( 'NONE',  ( 5.649999999999987921, 244.5000000000000000, 2.500000000000000000 ) ) ;
#19498=VERTEX_POINT ( 'NONE', #278 ) ;
#19526=VERTEX_POINT ( 'NONE', #20764 ) ;
#19576=ORIENTED_EDGE ( 'NONE', *, *, #19844, .T. ) ;
#19645=DIRECTION ( 'NONE',  ( 1.000000000000000000, 0.000000000000000000, 0.000000000000000000 ) ) ;
#19658=LINE ( 'NONE', #11293, #17467 ) ;
#19670=FACE_OUTER_BOUND ( 'NONE', #10126, .T. ) ;
#19684=ORIENTED_EDGE ( 'NONE', *, *, #34158, .T. ) ;
#19710=DIRECTION ( 'NONE',  ( 1.000000000000000000, 0.000000000000000000, 0.000000000000000000 ) ) ;
#19755=CARTESIAN_POINT ( 'NONE',  ( 10.49999999999999822, 252.0000000000000000, -2.499999999999986677 ) ) ;
#19765=EDGE_CURVE ( 'NONE', #25296, #19526, #31475, .T. ) ;
#19776=VERTEX_POINT ( 'NONE', #26384 ) ;
#19787=DIRECTION ( 'NONE',  ( -0.000000000000000000, 0.000000000000000000, 1.000000000000000000 ) ) ;
#19795=FACE_OUTER_BOUND ( 'NONE', #37196, .T. ) ;
#19809=DIRECTION ( 'NONE',  ( -0.000000000000000000, 1.000000000000000000, -0.000000000000000000 ) ) ;
#19844=EDGE_CURVE ( 'NONE', #19526, #7363, #26036, .T. ) ;
#19852=DIRECTION ( 'NONE',  ( 0.000000000000000000, 0.000000000000000000, 1.000000000000000000 ) ) ;
#19918=EDGE_CURVE ( 'NONE', #16035, #25296, #7252, .T. ) ;
#19954=ORIENTED_EDGE ( 'NONE', *, *, #8299, .T. ) ;
#20032=VERTEX_POINT ( 'NONE', #21481 ) ;
#20125=VERTEX_POINT ( 'NONE', #35668 ) ;
#20158=PLANE ( 'NONE',  #23479 ) ;
#20167=DIRECTION ( 'NONE',  ( -0.000000000000000000, 0.000000000000000000, 1.000000000000000000 ) ) ;
#20169=ORIENTED_EDGE ( 'NONE', *, *, #15827, .T. ) ;
#20227=LINE ( 'NONE', #23623, #30947 ) ;
#20229=CARTESIAN_POINT ( 'NONE',  ( -47.00000000000000711, 237.0000000000000000, 2.500000000000001776 ) ) ;
#20231=MANIFOLD_SOLID_BREP ( 'M5 Clearance Hole1', #34394 ) ;
#20246=CIRCLE ( 'NONE', #7529, 7.500000000000000000 ) ;
#20315=ORIENTED_EDGE ( 'NONE', *, *, #13660, .F. ) ;
#20375=ADVANCED_FACE ( 'NONE', ( #16538 ), #36420, .F. ) ;
#20405=ORIENTED_EDGE ( 'NONE', *, *, #31634, .T. ) ;
#20425=AXIS2_PLACEMENT_3D ( 'NONE', #36632, #28107, #13901 ) ;
#20447=CARTESIAN_POINT ( 'NONE',  ( 10.49999999999999645, 237.0000000000000000, 5.000000000000000000 ) ) ;
#20464=ORIENTED_EDGE ( 'NONE', *, *, #10991, .T. ) ;
#20511=CARTESIAN_POINT ( 'NONE',  ( -47.00000000000000711, 237.0000000000000000, 5.000000000000000000 ) ) ;
#20588=EDGE_LOOP ( 'NONE', ( #35154, #24545, #1222, #27022, #16742, #29861, #12825, #3, #37466, #10620, #11266, #14738 ) ) ;
#20596=DIRECTION ( 'NONE',  ( -2.057406622567553763E-16, 0.000000000000000000, 1.000000000000000000 ) ) ;
#20599=ORIENTED_EDGE ( 'NONE', *, *, #34724, .F. ) ;
#20628=DIRECTION ( 'NONE',  ( 1.000000000000000000, 0.000000000000000000, 0.000000000000000000 ) ) ;
#20721=EDGE_CURVE ( 'NONE', #9774, #23018, #12119, .T. ) ;
#20747=SURFACE_SIDE_STYLE ('',( #18474 ) ) ;
#20764=CARTESIAN_POINT ( 'NONE',  ( -54.50000000000000711, 244.5000000000000000, -5.000000000000000000 ) ) ;
#20789=CARTESIAN_POINT ( 'NONE',  ( -47.00000000000000711, 244.5000000000000000, 2.500000000000001776 ) ) ;
#20809=ADVANCED_FACE ( 'NONE', ( #13070, #24809 ), #16480, .T. ) ;
#20816=CARTESIAN_POINT ( 'NONE',  ( -47.00000000000000711, 244.5000000000000000, 5.000000000000000000 ) ) ;
#20853=CARTESIAN_POINT ( 'NONE',  ( 2.999999999999997335, 244.5000000000000000, 2.500000000000000000 ) ) ;
#20863=LINE ( 'NONE', #1123, #7364 ) ;
#21002=ORIENTED_EDGE ( 'NONE', *, *, #2188, .F. ) ;
#21012=DIRECTION ( 'NONE',  ( -1.000000000000000000, 0.000000000000000000, 0.000000000000000000 ) ) ;
#21019=CARTESIAN_POINT ( 'NONE',  ( -44.35000000000002274, 244.5000000000000000, 5.000000000000000888 ) ) ;
#21059=ORIENTED_EDGE ( 'NONE', *, *, #21920, .T. ) ;
#21190=ADVANCED_FACE ( 'NONE', ( #12648 ), #5275, .F. ) ;
#21285=ADVANCED_FACE ( 'NONE', ( #4206 ), #36043, .T. ) ;
#21374=ORIENTED_EDGE ( 'NONE', *, *, #18146, .T. ) ;
#21391=FACE_OUTER_BOUND ( 'NONE', #5961, .T. ) ;
#21402=ORIENTED_EDGE ( 'NONE', *, *, #7744, .F. ) ;
#21430=AXIS2_PLACEMENT_3D ( 'NONE', #10274, #19390, #7255 ) ;
#21481=CARTESIAN_POINT ( 'NONE',  ( -29.50000000000000711, 252.0000000000000000, -2.499999999999994671 ) ) ;
#21587=AXIS2_PLACEMENT_3D ( 'NONE', #27432, #27812, #36328 ) ;
#21597=CIRCLE ( 'NONE', #7062, 7.500000000000000000 ) ;
#21618=AXIS2_PLACEMENT_3D ( 'NONE', #13247, #27646, #4701 ) ;
#21634=ORIENTED_EDGE ( 'NONE', *, *, #36365, .F. ) ;
#21700=CIRCLE ( 'NONE', #31376, 7.500000000000000000 ) ;
#21706=CARTESIAN_POINT ( 'NONE',  ( -47.00000000000000711, 244.5000000000000000, 5.000000000000000000 ) ) ;
#21819=CARTESIAN_POINT ( 'NONE',  ( -47.00000000000000711, 244.5000000000000000, -2.499999999999997780 ) ) ;
#21881=CIRCLE ( 'NONE', #23690, 2.649999999999985700 ) ;
#21882=VERTEX_POINT ( 'NONE', #9814 ) ;
#21889=ADVANCED_FACE ( 'NONE', ( #21391 ), #32933, .T. ) ;
#21920=EDGE_CURVE ( 'NONE', #3698, #22652, #22789, .T. ) ;
#21929=ADVANCED_FACE ( 'NONE', ( #1273 ), #7354, .F. ) ;
#22014=EDGE_CURVE ( 'NONE', #23018, #20125, #25729, .T. ) ;
#22055=PRODUCT_DEFINITION_FORMATION_WITH_SPECIFIED_SOURCE ( 'ANY', '', #23177, .NOT_KNOWN. ) ;
#22063=PLANE ( 'NONE',  #20425 ) ;
#22116=VERTEX_POINT ( 'NONE', #19485 ) ;
#22168=CARTESIAN_POINT ( 'NONE',  ( 2.999999999999997335, 244.5000000000000000, 2.500000000000000000 ) ) ;
#22213=CIRCLE ( 'NONE', #21618, 2.649999999999994582 ) ;
#22241=CIRCLE ( 'NONE', #8907, 7.500000000000000000 ) ;
#22374=EDGE_LOOP ( 'NONE', ( #1099, #13552, #1162, #27075 ) ) ;
#22415=VECTOR ( 'NONE', #11434, 1000.000000000000000 ) ;
#22436=AXIS2_PLACEMENT_3D ( 'NONE', #2175, #13376, #13757 ) ;
#22503=DIRECTION ( 'NONE',  ( -0.000000000000000000, -0.000000000000000000, 1.000000000000000000 ) ) ;
#22562=DIRECTION ( 'NONE',  ( 2.057406622567553763E-16, -0.000000000000000000, -1.000000000000000000 ) ) ;
#22601=MECHANICAL_DESIGN_GEOMETRIC_PRESENTATION_REPRESENTATION('',(#6872),#32865);
#22652=VERTEX_POINT ( 'NONE', #29999 ) ;
#22758=CARTESIAN_POINT ( 'NONE',  ( 2.999999999999997335, 244.5000000000000000, 5.000000000000000000 ) ) ;
#22789=CIRCLE ( 'NONE', #33061, 7.500000000000000000 ) ;
#22811=CARTESIAN_POINT ( 'NONE',  ( 0.000000000000000000, 0.000000000000000000, -5.000000000000000000 ) ) ;
#22829=VERTEX_POINT ( 'NONE', #7176 ) ;
#22958=VERTEX_POINT ( 'NONE', #1472 ) ;
#22995=CARTESIAN_POINT ( 'NONE',  ( -47.00000000000000711, 244.5000000000000000, -5.000000000000000000 ) ) ;
#22999=FACE_BOUND ( 'NONE', #26452, .T. ) ;
#23018=VERTEX_POINT ( 'NONE', #30485 ) ;
#23040=EDGE_LOOP ( 'NONE', ( #28115, #5877, #32279, #34250 ) ) ;
#23047=MECHANICAL_DESIGN_GEOMETRIC_PRESENTATION_REPRESENTATION('',(#30921),#9107);
#23096=DIRECTION ( 'NONE',  ( 0.000000000000000000, -0.000000000000000000, -1.000000000000000000 ) ) ;
#23097=EDGE_CURVE ( 'NONE', #8415, #20125, #2403, .T. ) ;
#23177=PRODUCT ( 'handle link', 'handle link', '', ( #27408 ) ) ;
#23195=DIRECTION ( 'NONE',  ( 1.000000000000000000, 0.000000000000000000, 0.000000000000000000 ) ) ;
#23251=AXIS2_PLACEMENT_3D ( 'NONE', #11115, #8279, #19852 ) ;
#23324=ORIENTED_EDGE ( 'NONE', *, *, #13888, .F. ) ;
#23362=EDGE_CURVE ( 'NONE', #21882, #8395, #7588, .T. ) ;
#23366=DIRECTION ( 'NONE',  ( 1.000000000000000000, 0.000000000000000000, 0.000000000000000000 ) ) ;
#23453=ORIENTED_EDGE ( 'NONE', *, *, #4065, .F. ) ;
#23455=CARTESIAN_POINT ( 'NONE',  ( -49.64999999999999858, 244.5000000000000000, 5.000000000000000000 ) ) ;
#23479=AXIS2_PLACEMENT_3D ( 'NONE', #31706, #5734, #14462 ) ;
#23575=ORIENTED_EDGE ( 'NONE', *, *, #29347, .F. ) ;
#23623=CARTESIAN_POINT ( 'NONE',  ( 10.49999999999999467, 237.0000000000000000, 2.500000000000000000 ) ) ;
#23662=CARTESIAN_POINT ( 'NONE',  ( 0.3500000000000100253, 244.5000000000000000, 5.000000000000000888 ) ) ;
#23665=DIRECTION ( 'NONE',  ( -0.000000000000000000, 0.000000000000000000, 1.000000000000000000 ) ) ;
#23670=ORIENTED_EDGE ( 'NONE', *, *, #35754, .T. ) ;
#23690=AXIS2_PLACEMENT_3D ( 'NONE', #6814, #29559, #3597 ) ;
#23750=DIRECTION ( 'NONE',  ( -1.000000000000000000, 0.000000000000000000, -0.000000000000000000 ) ) ;
#23813=COLOUR_RGB ( '',0.8941176470588234615, 0.8941176470588234615, 0.8941176470588234615 ) ;
#23845=DIRECTION ( 'NONE',  ( -0.000000000000000000, -0.000000000000000000, 1.000000000000000000 ) ) ;
#23857=LINE ( 'NONE', #27760, #15034 ) ;
#23869=VECTOR ( 'NONE', #33677, 1000.000000000000000 ) ;
#23886=CARTESIAN_POINT ( 'NONE',  ( 5.649999999999987921, 244.5000000000000000, 5.000000000000000000 ) ) ;
#23946=VECTOR ( 'NONE', #34056, 1000.000000000000000 ) ;
#23954=AXIS2_PLACEMENT_3D ( 'NONE', #14861, #34756, #32283 ) ;
#24032=CARTESIAN_POINT ( 'NONE',  ( -14.50000000000000355, 252.0000000000000000, 5.000000000000000000 ) ) ;
#24098=ORIENTED_EDGE ( 'NONE', *, *, #36365, .T. ) ;
#24112=DIRECTION ( 'NONE',  ( 1.000000000000000000, 0.000000000000000000, 0.000000000000000000 ) ) ;
#24131=CARTESIAN_POINT ( 'NONE',  ( -47.00000000000000711, 244.5000000000000000, 5.000000000000000000 ) ) ;
#24289=EDGE_CURVE ( 'NONE', #36103, #36641, #7001, .T. ) ;
#24320=FACE_OUTER_BOUND ( 'NONE', #2630, .T. ) ;
#24370=ORIENTED_EDGE ( 'NONE', *, *, #17296, .F. ) ;
#24419=VECTOR ( 'NONE', #12644, 1000.000000000000000 ) ;
#24441=DIRECTION ( 'NONE',  ( -1.000000000000000000, 0.000000000000000000, 0.000000000000000000 ) ) ;
#24545=ORIENTED_EDGE ( 'NONE', *, *, #29347, .T. ) ;
#24614=AXIS2_PLACEMENT_3D ( 'NONE', #11006, #8174, #14596 ) ;
#24627=FACE_OUTER_BOUND ( 'NONE', #10259, .T. ) ;
#24693=AXIS2_PLACEMENT_3D ( 'NONE', #10647, #13877, #25426 ) ;
#24725=ORIENTED_EDGE ( 'NONE', *, *, #1013, .F. ) ;
#24759=CARTESIAN_POINT ( 'NONE',  ( -47.00000000000000711, 252.0000000000000000, 5.000000000000000000 ) ) ;
#24778=DIRECTION ( 'NONE',  ( 0.000000000000000000, -0.000000000000000000, -1.000000000000000000 ) ) ;
#24809=FACE_OUTER_BOUND ( 'NONE', #8154, .T. ) ;
#24810=VECTOR ( 'NONE', #6988, 1000.000000000000000 ) ;
#24822=CYLINDRICAL_SURFACE ( 'NONE', #15634, 2.649999999999992806 ) ;
#24873=EDGE_LOOP ( 'NONE', ( #13933, #25798 ) ) ;
#24919=ORIENTED_EDGE ( 'NONE', *, *, #13623, .F. ) ;
#25006=DIRECTION ( 'NONE',  ( 1.000000000000000000, 0.000000000000000000, 2.312964634635742957E-16 ) ) ;
#25070=( NAMED_UNIT ( * ) PLANE_ANGLE_UNIT ( ) SI_UNIT ( $, .RADIAN. ) );
#25296=VERTEX_POINT ( 'NONE', #3710 ) ;
#25365=CARTESIAN_POINT ( 'NONE',  ( -47.00000000000000711, 244.5000000000000000, 5.000000000000000000 ) ) ;
#25372=CARTESIAN_POINT ( 'NONE',  ( 2.999999999999997335, 244.5000000000000000, -5.000000000000001776 ) ) ;
#25413=EDGE_CURVE ( 'NONE', #14298, #30074, #30007, .T. ) ;
#25426=DIRECTION ( 'NONE',  ( 1.000000000000000000, 0.000000000000000000, 0.000000000000000000 ) ) ;
#25443=DIRECTION ( 'NONE',  ( -0.000000000000000000, 0.000000000000000000, 1.000000000000000000 ) ) ;
#25610=FACE_OUTER_BOUND ( 'NONE', #23040, .T. ) ;
#25612=CARTESIAN_POINT ( 'NONE',  ( 2.999999999999997335, 244.5000000000000000, 5.000000000000000000 ) ) ;
#25627=CARTESIAN_POINT ( 'NONE',  ( 2.999999999999997335, 244.5000000000000000, 2.500000000000000000 ) ) ;
#25630=DIRECTION ( 'NONE',  ( 1.000000000000000000, 0.000000000000000000, 0.000000000000000000 ) ) ;
#25633=CARTESIAN_POINT ( 'NONE',  ( 2.999999999999997335, 252.0000000000000000, 2.500000000000000000 ) ) ;
#25729=CIRCLE ( 'NONE', #17349, 2.649999999999991029 ) ;
#25798=ORIENTED_EDGE ( 'NONE', *, *, #10991, .F. ) ;
#25828=CARTESIAN_POINT ( 'NONE',  ( -47.00000000000000711, 244.5000000000000000, -5.000000000000000000 ) ) ;
#25857=EDGE_CURVE ( 'NONE', #19019, #12668, #3289, .T. ) ;
#25892=PRODUCT_DEFINITION_SHAPE ( 'NONE', 'NONE',  #10201 ) ;
#25903=ADVANCED_FACE ( 'NONE', ( #8800 ), #29248, .F. ) ;
#25960=CARTESIAN_POINT ( 'NONE',  ( -29.50000000000000711, 237.0000000000000000, -2.499999999999994671 ) ) ;
#25980=DIRECTION ( 'NONE',  ( 0.000000000000000000, 0.000000000000000000, 1.000000000000000000 ) ) ;
#25991=VERTEX_POINT ( 'NONE', #34938 ) ;
#26003=DIRECTION ( 'NONE',  ( 0.000000000000000000, 0.000000000000000000, 1.000000000000000000 ) ) ;
#26014=DIRECTION ( 'NONE',  ( 1.000000000000000000, 0.000000000000000000, 0.000000000000000000 ) ) ;
#26036=CIRCLE ( 'NONE', #11511, 7.500000000000000000 ) ;
#26044=EDGE_CURVE ( 'NONE', #20032, #18087, #5133, .T. ) ;
#26077=CARTESIAN_POINT ( 'NONE',  ( -47.00000000000000711, 244.5000000000000000, -5.000000000000001776 ) ) ;
#26234=VERTEX_POINT ( 'NONE', #28437 ) ;
#26269=PRODUCT_DEFINITION_CONTEXT ( 'detailed design', #28197, 'design' ) ;
#26288=LINE ( 'NONE', #23455, #24419 ) ;
#26384=CARTESIAN_POINT ( 'NONE',  ( -29.50000000000000711, 252.0000000000000000, 2.500000000000005329 ) ) ;
#26452=EDGE_LOOP ( 'NONE', ( #24370, #2884 ) ) ;
#26472=ORIENTED_EDGE ( 'NONE', *, *, #28486, .F. ) ;
#26635=CARTESIAN_POINT ( 'NONE',  ( -47.00000000000000711, 244.5000000000000000, 2.500000000000001776 ) ) ;
#26640=PLANE ( 'NONE',  #33450 ) ;
#26712=CARTESIAN_POINT ( 'NONE',  ( 10.49999999999999645, 237.0000000000000000, 5.000000000000000000 ) ) ;
#26729=ORIENTED_EDGE ( 'NONE', *, *, #34869, .F. ) ;
#26793=( NAMED_UNIT ( * ) SI_UNIT ( $, .STERADIAN. ) SOLID_ANGLE_UNIT ( ) );
#26794=CARTESIAN_POINT ( 'NONE',  ( -47.00000000000000711, 237.0000000000000000, -2.499999999999998224 ) ) ;
#26906=CARTESIAN_POINT ( 'NONE',  ( -54.50000000000000711, 237.0000000000000000, 2.500000000000000000 ) ) ;
#26939=CARTESIAN_POINT ( 'NONE',  ( 2.999999999999997335, 244.5000000000000000, 5.000000000000000888 ) ) ;
#26959=EDGE_CURVE ( 'NONE', #25991, #22829, #21597, .T. ) ;
#27022=ORIENTED_EDGE ( 'NONE', *, *, #9463, .F. ) ;
#27075=ORIENTED_EDGE ( 'NONE', *, *, #11087, .T. ) ;
#27099=DIRECTION ( 'NONE',  ( -2.057406622567553763E-16, 0.000000000000000000, 1.000000000000000000 ) ) ;
#27140=CARTESIAN_POINT ( 'NONE',  ( -14.50000000000000533, 237.0000000000000000, 2.500000000000000000 ) ) ;
#27165=EDGE_LOOP ( 'NONE', ( #2338, #10188, #2591, #11488, #8797, #18043, #35032, #30755, #27209, #20405, #561, #23670 ) ) ;
#27209=ORIENTED_EDGE ( 'NONE', *, *, #17535, .F. ) ;
#27276=FACE_OUTER_BOUND ( 'NONE', #10464, .T. ) ;
#27308=ORIENTED_EDGE ( 'NONE', *, *, #4065, .T. ) ;
#27344=VECTOR ( 'NONE', #6773, 1000.000000000000000 ) ;
#27392=ORIENTED_EDGE ( 'NONE', *, *, #37182, .F. ) ;
#27408=PRODUCT_CONTEXT ( 'NONE', #34708, 'mechanical' ) ;
#27432=CARTESIAN_POINT ( 'NONE',  ( 2.999999999999997335, 244.5000000000000000, 5.000000000000000000 ) ) ;
#27448=EDGE_CURVE ( 'NONE', #8594, #36641, #30920, .T. ) ;
#27553=CARTESIAN_POINT ( 'NONE',  ( -14.50000000000000533, 252.0000000000000000, 2.500000000000000000 ) ) ;
#27640=ADVANCED_FACE ( 'NONE', ( #11189 ), #10821, .T. ) ;
#27646=DIRECTION ( 'NONE',  ( -0.000000000000000000, -0.000000000000000000, 1.000000000000000000 ) ) ;
#27676=VERTEX_POINT ( 'NONE', #8536 ) ;
#27693=VECTOR ( 'NONE', #3301, 1000.000000000000000 ) ;
#27760=CARTESIAN_POINT ( 'NONE',  ( 2.999999999999997335, 252.0000000000000000, -5.000000000000000000 ) ) ;
#27770=CIRCLE ( 'NONE', #4765, 7.500000000000000000 ) ;
#27780=FACE_OUTER_BOUND ( 'NONE', #30623, .T. ) ;
#27812=DIRECTION ( 'NONE',  ( -0.000000000000000000, -0.000000000000000000, 1.000000000000000000 ) ) ;
#27840=VECTOR ( 'NONE', #11068, 1000.000000000000000 ) ;
#27934=DIRECTION ( 'NONE',  ( 0.000000000000000000, 0.000000000000000000, 1.000000000000000000 ) ) ;
#27994=ORIENTED_EDGE ( 'NONE', *, *, #13578, .F. ) ;
#28003=EDGE_LOOP ( 'NONE', ( #29606, #27308 ) ) ;
#28052=DIRECTION ( 'NONE',  ( 1.000000000000000000, 0.000000000000000000, 2.312964634635742957E-16 ) ) ;
#28104=AXIS2_PLACEMENT_3D ( 'NONE', #28953, #331, #21012 ) ;
#28107=DIRECTION ( 'NONE',  ( 0.000000000000000000, -1.000000000000000000, 0.000000000000000000 ) ) ;
#28115=ORIENTED_EDGE ( 'NONE', *, *, #29776, .F. ) ;
#28175=LINE ( 'NONE', #16815, #34726 ) ;
#28190=CIRCLE ( 'NONE', #31803, 7.500000000000000000 ) ;
#28197=APPLICATION_CONTEXT ( 'automotive_design' ) ;
#28216=DIRECTION ( 'NONE',  ( -0.000000000000000000, -0.000000000000000000, 1.000000000000000000 ) ) ;
#28222=ORIENTED_EDGE ( 'NONE', *, *, #24289, .T. ) ;
#28262=VERTEX_POINT ( 'NONE', #12676 ) ;
#28272=ORIENTED_EDGE ( 'NONE', *, *, #29776, .T. ) ;
#28286=DIRECTION ( 'NONE',  ( -1.000000000000000000, 0.000000000000000000, 0.000000000000000000 ) ) ;
#28437=CARTESIAN_POINT ( 'NONE',  ( -14.50000000000000533, 252.0000000000000000, -2.500000000000000000 ) ) ;
#28486=EDGE_CURVE ( 'NONE', #8415, #9774, #22213, .T. ) ;
#28487=LINE ( 'NONE', #28858, #22415 ) ;
#28632=CARTESIAN_POINT ( 'NONE',  ( -47.00000000000000711, 244.5000000000000000, 5.000000000000000000 ) ) ;
#28668=DIRECTION ( 'NONE',  ( 0.000000000000000000, 0.000000000000000000, -1.000000000000000000 ) ) ;
#28675=DIRECTION ( 'NONE',  ( -0.000000000000000000, 1.000000000000000000, -0.000000000000000000 ) ) ;
#28726=ORIENTED_EDGE ( 'NONE', *, *, #11552, .T. ) ;
#28786=FACE_OUTER_BOUND ( 'NONE', #33622, .T. ) ;
#28815=DIRECTION ( 'NONE',  ( 1.000000000000000000, 0.000000000000000000, 2.312964634635742957E-16 ) ) ;
#28821=ORIENTED_EDGE ( 'NONE', *, *, #26044, .T. ) ;
#28853=AXIS2_PLACEMENT_3D ( 'NONE', #2509, #26003, #25630 ) ;
#28857=CARTESIAN_POINT ( 'NONE',  ( -47.00000000000000711, 244.5000000000000000, 5.000000000000000888 ) ) ;
#28858=CARTESIAN_POINT ( 'NONE',  ( 10.49999999999999645, 252.0000000000000000, -5.000000000000000000 ) ) ;
#28896=ORIENTED_EDGE ( 'NONE', *, *, #1013, .T. ) ;
#28913=ORIENTED_EDGE ( 'NONE', *, *, #37247, .T. ) ;
#28953=CARTESIAN_POINT ( 'NONE',  ( 2.999999999999997335, 244.5000000000000000, 2.500000000000000000 ) ) ;
#29044=LINE ( 'NONE', #37208, #19034 ) ;
#29055=AXIS2_PLACEMENT_3D ( 'NONE', #25612, #8375, #10463 ) ;
#29084=ADVANCED_FACE ( 'NONE', ( #1245 ), #3907, .F. ) ;
#29101=DIRECTION ( 'NONE',  ( -0.000000000000000000, -0.000000000000000000, 1.000000000000000000 ) ) ;
#29135=CARTESIAN_POINT ( 'NONE',  ( 10.49999999999999645, 244.5000000000000000, 5.000000000000000000 ) ) ;
#29248=CYLINDRICAL_SURFACE ( 'NONE', #23954, 2.649999999999991029 ) ;
#29326=CARTESIAN_POINT ( 'NONE',  ( 2.999999999999997335, 252.0000000000000000, -5.000000000000000000 ) ) ;
#29327=CARTESIAN_POINT ( 'NONE',  ( -44.35000000000001563, 244.5000000000000000, 5.000000000000000000 ) ) ;
#29347=EDGE_CURVE ( 'NONE', #19776, #19019, #2131, .T. ) ;
#29396=AXIS2_PLACEMENT_3D ( 'NONE', #26077, #8464, #34427 ) ;
#29442=CARTESIAN_POINT ( 'NONE',  ( -47.00000000000000711, 252.0000000000000000, 5.000000000000000000 ) ) ;
#29559=DIRECTION ( 'NONE',  ( -0.000000000000000000, -0.000000000000000000, 1.000000000000000000 ) ) ;
#29571=DIRECTION ( 'NONE',  ( -0.000000000000000000, 0.000000000000000000, 1.000000000000000000 ) ) ;
#29606=ORIENTED_EDGE ( 'NONE', *, *, #22014, .T. ) ;
#29776=EDGE_CURVE ( 'NONE', #35447, #19526, #31556, .T. ) ;
#29786=ORIENTED_EDGE ( 'NONE', *, *, #5674, .T. ) ;
#29861=ORIENTED_EDGE ( 'NONE', *, *, #35826, .F. ) ;
#29863=DIRECTION ( 'NONE',  ( 0.000000000000000000, 0.000000000000000000, -1.000000000000000000 ) ) ;
#29982=LINE ( 'NONE', #27140, #17637 ) ;
#29999=CARTESIAN_POINT ( 'NONE',  ( 10.49999999999999645, 244.5000000000000000, -5.000000000000000000 ) ) ;
#30007=CIRCLE ( 'NONE', #34256, 2.649999999999992806 ) ;
#30027=CARTESIAN_POINT ( 'NONE',  ( -47.00000000000000711, 252.0000000000000000, 5.000000000000000000 ) ) ;
#30043=VECTOR ( 'NONE', #16519, 1000.000000000000000 ) ;
#30074=VERTEX_POINT ( 'NONE', #35697 ) ;
#30127=CARTESIAN_POINT ( 'NONE',  ( -54.50000000000000711, 237.0000000000000000, -2.500000000000000000 ) ) ;
#30177=UNCERTAINTY_MEASURE_WITH_UNIT (LENGTH_MEASURE( 1.000000000000000082E-05 ), #6522, 'distance_accuracy_value', 'NONE');
#30240=VERTEX_POINT ( 'NONE', #16374 ) ;
#30273=ADVANCED_FACE ( 'NONE', ( #2330 ), #22063, .F. ) ;
#30313=DIRECTION ( 'NONE',  ( 1.000000000000000000, 0.000000000000000000, 0.000000000000000000 ) ) ;
#30347=VERTEX_POINT ( 'NONE', #27553 ) ;
#30485=CARTESIAN_POINT ( 'NONE',  ( 5.649999999999987921, 244.5000000000000000, -2.499999999999999556 ) ) ;
#30489=VERTEX_POINT ( 'NONE', #25633 ) ;
#30508=CARTESIAN_POINT ( 'NONE',  ( -47.00000000000000711, 244.5000000000000000, 5.000000000000000000 ) ) ;
#30524=CARTESIAN_POINT ( 'NONE',  ( -47.00000000000000711, 244.5000000000000000, 5.000000000000000000 ) ) ;
#30533=FACE_BOUND ( 'NONE', #28003, .T. ) ;
#30538=LINE ( 'NONE', #4923, #7110 ) ;
#30559=EDGE_CURVE ( 'NONE', #19776, #20032, #30538, .T. ) ;
#30560=CARTESIAN_POINT ( 'NONE',  ( 2.999999999999997335, 237.0000000000000000, -2.500000000000000000 ) ) ;
#30573=EDGE_CURVE ( 'NONE', #35447, #18087, #22241, .T. ) ;
#30623=EDGE_LOOP ( 'NONE', ( #28726, #32973, #14951, #1938, #17141, #783 ) ) ;
#30692=LINE ( 'NONE', #4709, #1385 ) ;
#30744=EDGE_LOOP ( 'NONE', ( #16539, #3191, #13554, #27392 ) ) ;
#30755=ORIENTED_EDGE ( 'NONE', *, *, #2683, .F. ) ;
#30907=AXIS2_PLACEMENT_3D ( 'NONE', #22168, #16853, #31063 ) ;
#30920=LINE ( 'NONE', #4937, #30043 ) ;
#30921=STYLED_ITEM('',(#37556),#20231);
#30947=VECTOR ( 'NONE', #9029, 1000.000000000000000 ) ;
#30949=UNCERTAINTY_MEASURE_WITH_UNIT (LENGTH_MEASURE( 1.000000000000000082E-05 ), #7623, 'distance_accuracy_value', 'NONE');
#30983=CARTESIAN_POINT ( 'NONE',  ( -54.50000000000000711, 237.0000000000000000, 2.500000000000000000 ) ) ;
#31063=DIRECTION ( 'NONE',  ( -1.000000000000000000, 0.000000000000000000, 0.000000000000000000 ) ) ;
#31114=ORIENTED_EDGE ( 'NONE', *, *, #15827, .F. ) ;
#31145=ORIENTED_EDGE ( 'NONE', *, *, #34158, .F. ) ;
#31201=DIRECTION ( 'NONE',  ( 1.000000000000000000, 0.000000000000000000, 2.057406622567553516E-16 ) ) ;
#31213=ORIENTED_EDGE ( 'NONE', *, *, #35754, .F. ) ;
#31295=EDGE_LOOP ( 'NONE', ( #13909, #21002 ) ) ;
#31323=ORIENTED_EDGE ( 'NONE', *, *, #23362, .T. ) ;
#31375=CARTESIAN_POINT ( 'NONE',  ( -54.50000000000000711, 244.5000000000000000, -5.000000000000000000 ) ) ;
#31376=AXIS2_PLACEMENT_3D ( 'NONE', #13172, #23665, #11907 ) ;
#31475=CIRCLE ( 'NONE', #32066, 7.500000000000000000 ) ;
#31488=VERTEX_POINT ( 'NONE', #15314 ) ;
#31538=EDGE_LOOP ( 'NONE', ( #27994, #31114, #18041, #14529 ) ) ;
#31556=LINE ( 'NONE', #31375, #27693 ) ;
#31634=EDGE_CURVE ( 'NONE', #30240, #22958, #28175, .T. ) ;
#31666=DIRECTION ( 'NONE',  ( 2.057406622567553763E-16, -0.000000000000000000, -1.000000000000000000 ) ) ;
#31706=CARTESIAN_POINT ( 'NONE',  ( 10.49999999999999467, 237.0000000000000000, 2.500000000000000000 ) ) ;
#31803=AXIS2_PLACEMENT_3D ( 'NONE', #32226, #29571, #18217 ) ;
#31866=ADVANCED_FACE ( 'NONE', ( #19670 ), #16445, .T. ) ;
#31879=CARTESIAN_POINT ( 'NONE',  ( 2.999999999999997335, 244.5000000000000000, -2.499999999999999556 ) ) ;
#31968=VECTOR ( 'NONE', #13836, 1000.000000000000000 ) ;
#31982=DIRECTION ( 'NONE',  ( -0.000000000000000000, 0.000000000000000000, 1.000000000000000000 ) ) ;
#32066=AXIS2_PLACEMENT_3D ( 'NONE', #22995, #14646, #23366 ) ;
#32175=DIRECTION ( 'NONE',  ( -0.000000000000000000, -0.000000000000000000, 1.000000000000000000 ) ) ;
#32226=CARTESIAN_POINT ( 'NONE',  ( 2.999999999999997335, 244.5000000000000000, 5.000000000000000000 ) ) ;
#32279=ORIENTED_EDGE ( 'NONE', *, *, #746, .F. ) ;
#32283=DIRECTION ( 'NONE',  ( 1.000000000000000000, 0.000000000000000000, 0.000000000000000000 ) ) ;
#32455=FACE_OUTER_BOUND ( 'NONE', #17779, .T. ) ;
#32503=CARTESIAN_POINT ( 'NONE',  ( -47.00000000000000711, 252.0000000000000000, -5.000000000000000000 ) ) ;
#32691=VECTOR ( 'NONE', #3778, 1000.000000000000000 ) ;
#32771=DIRECTION ( 'NONE',  ( 0.000000000000000000, -0.000000000000000000, -1.000000000000000000 ) ) ;
#32779=PLANE ( 'NONE',  #18862 ) ;
#32804=CARTESIAN_POINT ( 'NONE',  ( 10.49999999999999645, 244.5000000000000000, 5.000000000000000000 ) ) ;
#32828=CARTESIAN_POINT ( 'NONE',  ( -47.00000000000000711, 237.0000000000000000, 5.000000000000000000 ) ) ;
#32852=FILL_AREA_STYLE ('',( #35507 ) ) ;
#32865=( GEOMETRIC_REPRESENTATION_CONTEXT ( 3 ) GLOBAL_UNCERTAINTY_ASSIGNED_CONTEXT ( ( #15782 ) ) GLOBAL_UNIT_ASSIGNED_CONTEXT ( ( #10665, #25070, #10853 ) ) REPRESENTATION_CONTEXT ( 'NONE', 'WORKASPACE' ) );
#32933=CYLINDRICAL_SURFACE ( 'NONE', #1587, 7.500000000000000000 ) ;
#32953=VECTOR ( 'NONE', #23845, 1000.000000000000000 ) ;
#32973=ORIENTED_EDGE ( 'NONE', *, *, #11274, .T. ) ;
#33061=AXIS2_PLACEMENT_3D ( 'NONE', #9998, #24778, #4680 ) ;
#33119=FACE_OUTER_BOUND ( 'NONE', #22374, .T. ) ;
#33141=DIRECTION ( 'NONE',  ( 0.000000000000000000, 0.000000000000000000, -1.000000000000000000 ) ) ;
#33173=CARTESIAN_POINT ( 'NONE',  ( -47.00000000000000711, 244.5000000000000000, -2.499999999999997780 ) ) ;
#33256=DIRECTION ( 'NONE',  ( -1.000000000000000000, 0.000000000000000000, 0.000000000000000000 ) ) ;
#33261=ORIENTED_EDGE ( 'NONE', *, *, #6855, .T. ) ;
#33314=DIRECTION ( 'NONE',  ( 0.000000000000000000, 0.000000000000000000, 1.000000000000000000 ) ) ;
#33344=DIRECTION ( 'NONE',  ( -2.057406622567553763E-16, 0.000000000000000000, 1.000000000000000000 ) ) ;
#33450=AXIS2_PLACEMENT_3D ( 'NONE', #8341, #29863, #35354 ) ;
#33550=AXIS2_PLACEMENT_3D ( 'NONE', #8786, #20167, #23195 ) ;
#33622=EDGE_LOOP ( 'NONE', ( #3945, #26729, #14474, #36370, #14483 ) ) ;
#33664=ORIENTED_EDGE ( 'NONE', *, *, #21920, .F. ) ;
#33677=DIRECTION ( 'NONE',  ( -0.000000000000000000, -0.000000000000000000, 1.000000000000000000 ) ) ;
#33690=ADVANCED_FACE ( 'NONE', ( #22999, #34548 ), #20158, .T. ) ;
#33731=DIRECTION ( 'NONE',  ( -0.000000000000000000, -0.000000000000000000, 1.000000000000000000 ) ) ;
#33831=ORIENTED_EDGE ( 'NONE', *, *, #14204, .F. ) ;
#33897=DIRECTION ( 'NONE',  ( -0.000000000000000000, 0.000000000000000000, 1.000000000000000000 ) ) ;
#33932=CIRCLE ( 'NONE', #10935, 2.649999999999992806 ) ;
#34056=DIRECTION ( 'NONE',  ( -0.000000000000000000, -0.000000000000000000, 1.000000000000000000 ) ) ;
#34074=AXIS2_PLACEMENT_3D ( 'NONE', #4156, #33344, #15726 ) ;
#34158=EDGE_CURVE ( 'NONE', #35111, #19498, #462, .T. ) ;
#34233=LINE ( 'NONE', #13595, #23869 ) ;
#34250=ORIENTED_EDGE ( 'NONE', *, *, #19844, .F. ) ;
#34256=AXIS2_PLACEMENT_3D ( 'NONE', #6947, #9963, #7315 ) ;
#34328=CYLINDRICAL_SURFACE ( 'NONE', #18806, 7.500000000000000000 ) ;
#34394=CLOSED_SHELL ( 'NONE', ( #21929, #17111, #29084, #21190, #15140, #8902, #21889, #21285, #30273, #37390, #15907, #2707, #27640, #11008, #2308, #9384, #10779, #10109, #33690, #31866, #2051, #20809, #9509, #34828, #20375, #25903 ) ) ;
#34427=DIRECTION ( 'NONE',  ( 1.000000000000000000, 0.000000000000000000, 0.000000000000000000 ) ) ;
#34432=CARTESIAN_POINT ( 'NONE',  ( 0.3500000000000065281, 244.5000000000000000, 5.000000000000000000 ) ) ;
#34519=AXIS2_PLACEMENT_3D ( 'NONE', #25627, #25443, #28286 ) ;
#34548=FACE_OUTER_BOUND ( 'NONE', #16263, .T. ) ;
#34656=ORIENTED_EDGE ( 'NONE', *, *, #37146, .T. ) ;
#34671=VECTOR ( 'NONE', #32175, 1000.000000000000000 ) ;
#34683=DIRECTION ( 'NONE',  ( -1.000000000000000000, 0.000000000000000000, -2.057406622567553763E-16 ) ) ;
#34704=ORIENTED_EDGE ( 'NONE', *, *, #19765, .T. ) ;
#34708=APPLICATION_CONTEXT ( 'automotive_design' ) ;
#34724=EDGE_CURVE ( 'NONE', #16035, #35447, #5927, .T. ) ;
#34726=VECTOR ( 'NONE', #22503, 1000.000000000000000 ) ;
#34735=CYLINDRICAL_SURFACE ( 'NONE', #17064, 7.500000000000000000 ) ;
#34756=DIRECTION ( 'NONE',  ( -0.000000000000000000, -0.000000000000000000, 1.000000000000000000 ) ) ;
#34813=AXIS2_PLACEMENT_3D ( 'NONE', #26635, #20596, #35542 ) ;
#34828=ADVANCED_FACE ( 'NONE', ( #13456 ), #24822, .F. ) ;
#34869=EDGE_CURVE ( 'NONE', #18512, #28262, #16120, .T. ) ;
#34938=CARTESIAN_POINT ( 'NONE',  ( 10.49999999999999467, 244.5000000000000000, -2.500000000000000000 ) ) ;
#35017=DIRECTION ( 'NONE',  ( -0.000000000000000000, -0.000000000000000000, 1.000000000000000000 ) ) ;
#35027=DIRECTION ( 'NONE',  ( 0.000000000000000000, 0.000000000000000000, -1.000000000000000000 ) ) ;
#35032=ORIENTED_EDGE ( 'NONE', *, *, #34869, .T. ) ;
#35111=VERTEX_POINT ( 'NONE', #2625 ) ;
#35123=DIRECTION ( 'NONE',  ( -0.000000000000000000, -0.000000000000000000, 1.000000000000000000 ) ) ;
#35154=ORIENTED_EDGE ( 'NONE', *, *, #30559, .F. ) ;
#35272=ORIENTED_EDGE ( 'NONE', *, *, #3200, .T. ) ;
#35354=DIRECTION ( 'NONE',  ( -1.000000000000000000, 0.000000000000000000, -0.000000000000000000 ) ) ;
#35373=EDGE_CURVE ( 'NONE', #18512, #25991, #21700, .T. ) ;
#35401=ORIENTED_EDGE ( 'NONE', *, *, #15360, .T. ) ;
#35419=EDGE_CURVE ( 'NONE', #27676, #30489, #23857, .T. ) ;
#35424=VECTOR ( 'NONE', #16904, 1000.000000000000000 ) ;
#35447=VERTEX_POINT ( 'NONE', #7303 ) ;
#35477=DIRECTION ( 'NONE',  ( -1.000000000000000000, 0.000000000000000000, 0.000000000000000000 ) ) ;
#35484=DIRECTION ( 'NONE',  ( -1.000000000000000000, 0.000000000000000000, -0.000000000000000000 ) ) ;
#35507=FILL_AREA_STYLE_COLOUR ( '', #23813 ) ;
#35527=DIRECTION ( 'NONE',  ( -0.000000000000000000, -0.000000000000000000, 1.000000000000000000 ) ) ;
#35542=DIRECTION ( 'NONE',  ( 1.000000000000000000, 0.000000000000000000, 1.636531581110199847E-16 ) ) ;
#35585=CIRCLE ( 'NONE', #4714, 2.649999999999987477 ) ;
#35613=CYLINDRICAL_SURFACE ( 'NONE', #12895, 7.500000000000000000 ) ;
#35617=DIRECTION ( 'NONE',  ( 1.000000000000000000, 0.000000000000000000, 0.000000000000000000 ) ) ;
#35668=CARTESIAN_POINT ( 'NONE',  ( 0.3500000000000065281, 244.5000000000000000, -2.499999999999999556 ) ) ;
#35697=CARTESIAN_POINT ( 'NONE',  ( -49.64999999999999858, 244.5000000000000000, -2.499999999999998224 ) ) ;
#35754=EDGE_CURVE ( 'NONE', #36846, #36103, #914, .T. ) ;
#35826=EDGE_CURVE ( 'NONE', #30347, #30489, #19319, .T. ) ;
#35929=DIRECTION ( 'NONE',  ( 1.000000000000000000, 0.000000000000000000, 0.000000000000000000 ) ) ;
#35943=DIRECTION ( 'NONE',  ( -0.000000000000000000, -0.000000000000000000, 1.000000000000000000 ) ) ;
#36043=CYLINDRICAL_SURFACE ( 'NONE', #36080, 7.500000000000000000 ) ;
#36080=AXIS2_PLACEMENT_3D ( 'NONE', #6492, #18066, #35477 ) ;
#36103=VERTEX_POINT ( 'NONE', #20229 ) ;
#36183=ORIENTED_EDGE ( 'NONE', *, *, #3543, .F. ) ;
#36279=CARTESIAN_POINT ( 'NONE',  ( -29.50000000000000711, 237.0000000000000000, 2.500000000000005329 ) ) ;
#36328=DIRECTION ( 'NONE',  ( 1.000000000000000000, 0.000000000000000000, 0.000000000000000000 ) ) ;
#36365=EDGE_CURVE ( 'NONE', #36641, #19019, #20246, .T. ) ;
#36370=ORIENTED_EDGE ( 'NONE', *, *, #26959, .T. ) ;
#36420=CYLINDRICAL_SURFACE ( 'NONE', #29055, 2.649999999999991029 ) ;
#36516=DIRECTION ( 'NONE',  ( 1.000000000000000000, 0.000000000000000000, 0.000000000000000000 ) ) ;
#36562=DIRECTION ( 'NONE',  ( 1.000000000000000000, 0.000000000000000000, 0.000000000000000000 ) ) ;
#36576=DIRECTION ( 'NONE',  ( 0.000000000000000000, 0.000000000000000000, -1.000000000000000000 ) ) ;
#36626=SURFACE_STYLE_USAGE ( .BOTH. , #20747 ) ;
#36632=CARTESIAN_POINT ( 'NONE',  ( 10.49999999999999645, 252.0000000000000000, 5.000000000000000000 ) ) ;
#36641=VERTEX_POINT ( 'NONE', #9964 ) ;
#36654=ORIENTED_EDGE ( 'NONE', *, *, #13623, .T. ) ;
#36709=LINE ( 'NONE', #10934, #23946 ) ;
#36783=EDGE_LOOP ( 'NONE', ( #31145, #10704, #20464, #1841 ) ) ;
#36846=VERTEX_POINT ( 'NONE', #20511 ) ;
#37056=DIRECTION ( 'NONE',  ( 1.000000000000000000, 0.000000000000000000, 0.000000000000000000 ) ) ;
#37113=VERTEX_POINT ( 'NONE', #32804 ) ;
#37146=EDGE_CURVE ( 'NONE', #18605, #22116, #1454, .T. ) ;
#37182=EDGE_CURVE ( 'NONE', #8395, #13579, #9434, .T. ) ;
#37195=PLANE ( 'NONE',  #19210 ) ;
#37196=EDGE_LOOP ( 'NONE', ( #18366, #34704, #19576, #33831, #21059, #882 ) ) ;
#37208=CARTESIAN_POINT ( 'NONE',  ( -29.50000000000000711, 237.0000000000000000, 2.500000000000005329 ) ) ;
#37247=EDGE_CURVE ( 'NONE', #31488, #37113, #3558, .T. ) ;
#37289=DIRECTION ( 'NONE',  ( 1.000000000000000000, 0.000000000000000000, 0.000000000000000000 ) ) ;
#37322=DIRECTION ( 'NONE',  ( 1.000000000000000000, 0.000000000000000000, 0.000000000000000000 ) ) ;
#37387=ORIENTED_EDGE ( 'NONE', *, *, #30559, .T. ) ;
#37390=ADVANCED_FACE ( 'NONE', ( #6018 ), #15311, .T. ) ;
#37466=ORIENTED_EDGE ( 'NONE', *, *, #6157, .T. ) ;
#37550=COLOUR_RGB('Off White',0.89,0.88,0.83);
#37551=FILL_AREA_STYLE_COLOUR('',#37550);
#37552=FILL_AREA_STYLE('',(#37551));
#37553=SURFACE_STYLE_FILL_AREA(#37552);
#37554=SURFACE_SIDE_STYLE('',(#37553));
#37555=SURFACE_STYLE_USAGE(.BOTH.,#37554);
#37556=PRESENTATION_STYLE_ASSIGNMENT((#37555));
ENDSEC;
END-ISO-10303-21;
